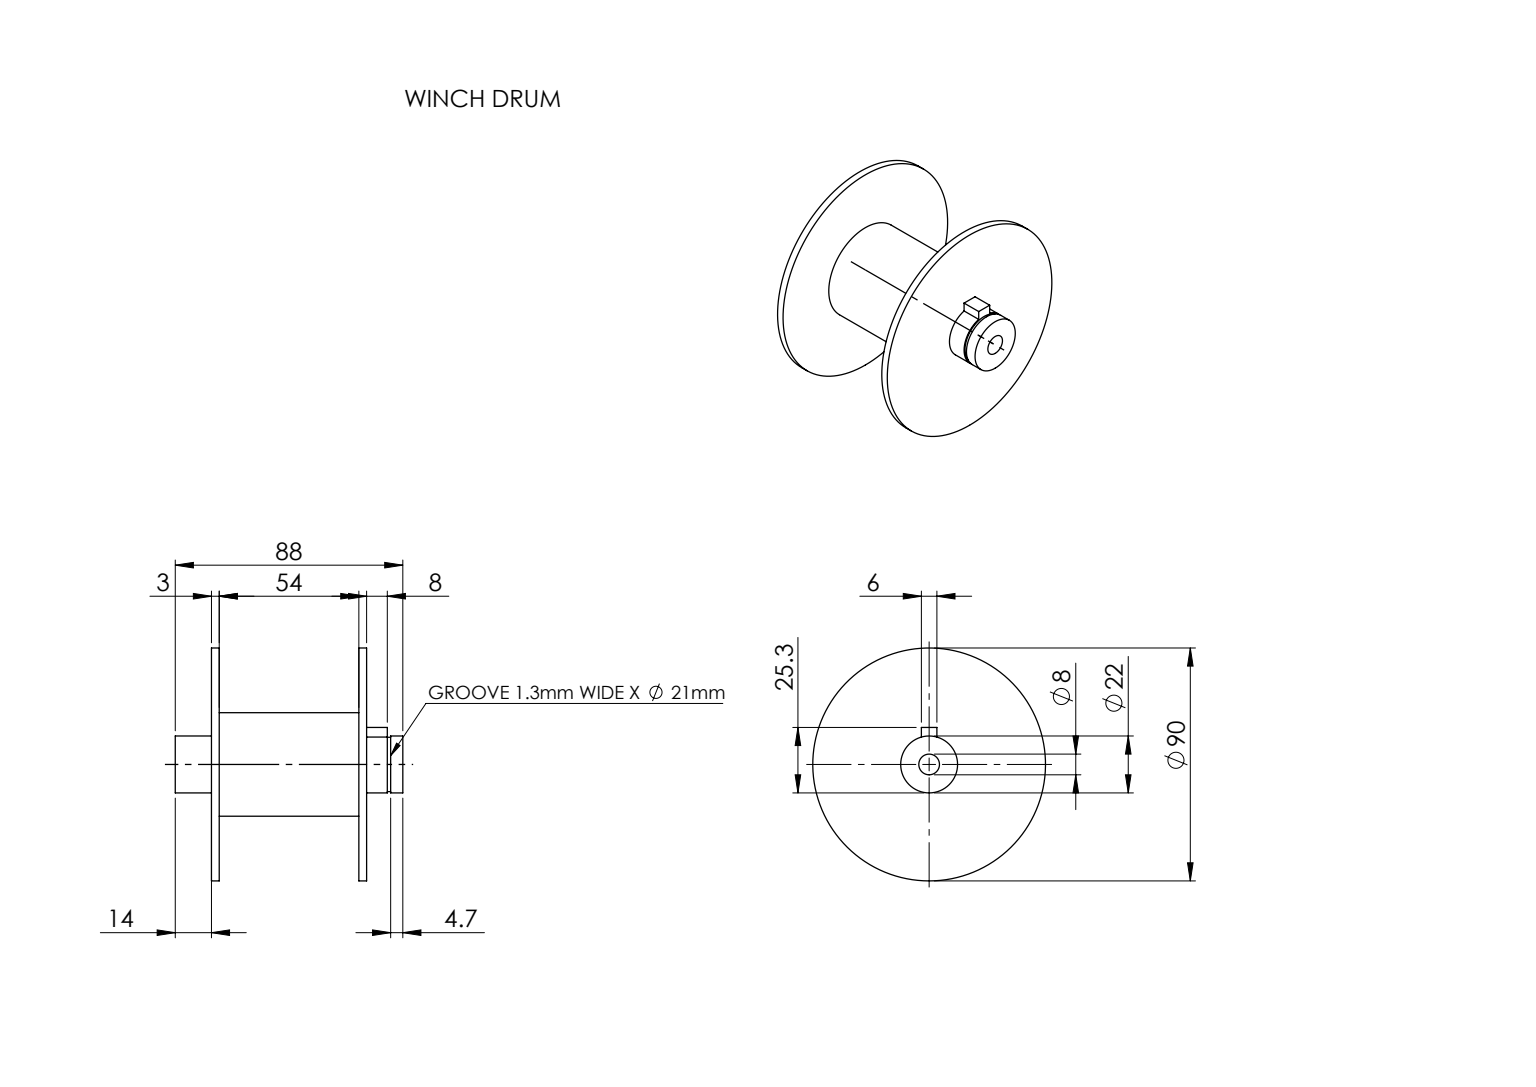
ISO-10303-21;
HEADER;
FILE_DESCRIPTION (('STEP AP214'),
    '1' );
FILE_NAME ('winch drum.step',
    '2026-09-28T15:49:00',
    ( '' ),
    ( '' ),
    'SwSTEP 2.0',
    'SolidWorks 2026',
    '' );
FILE_SCHEMA (( 'AUTOMOTIVE_DESIGN' ));
ENDSEC;

DATA;
#34=EDGE_CURVE ( 'NONE', #41, #24879, #23867, .T. ) ;
#41=VERTEX_POINT ( 'NONE', #30237 ) ;
#61=PRODUCT_DEFINITION_CONTEXT ( 'detailed design', #10343, 'design' ) ;
#131=DIRECTION ( 'NONE',  ( 3.154042683594195121E-16, -1.000000000000000000, 0.000000000000000000 ) ) ;
#150=CIRCLE ( 'NONE', #20253, 10.49999999999999645 ) ;
#165=EDGE_LOOP ( 'NONE', ( #34019, #14736, #9837, #7104, #34372 ) ) ;
#233=DIRECTION ( 'NONE',  ( 0.000000000000000000, 0.000000000000000000, -1.000000000000000000 ) ) ;
#284=CARTESIAN_POINT ( 'NONE',  ( 29.99999999999999289, 1.244980450007031636E-14, -3.000000000000002665 ) ) ;
#310=VECTOR ( 'NONE', #1724, 1000.000000000000000 ) ;
#429=DIRECTION ( 'NONE',  ( 0.000000000000000000, -1.000000000000000000, 0.000000000000000000 ) ) ;
#534=CYLINDRICAL_SURFACE ( 'NONE', #32662, 44.99999999999999289 ) ;
#567=ORIENTED_EDGE ( 'NONE', *, *, #16616, .F. ) ;
#653=CARTESIAN_POINT ( 'NONE',  ( 38.00000000000000000, -10.99999999999999112, 0.000000000000000000 ) ) ;
#680=DIRECTION ( 'NONE',  ( 1.000000000000000000, 1.836970198721029934E-16, 0.000000000000000000 ) ) ;
#700=DIRECTION ( 'NONE',  ( 1.541976423090495387E-16, -1.000000000000000000, 0.000000000000000000 ) ) ;
#729=ORIENTED_EDGE ( 'NONE', *, *, #32592, .F. ) ;
#737=CIRCLE ( 'NONE', #20844, 44.99999999999999289 ) ;
#790=DIRECTION ( 'NONE',  ( 1.734723475976807341E-16, -1.000000000000000000, 0.000000000000000000 ) ) ;
#808=DIRECTION ( 'NONE',  ( 1.000000000000000000, 1.836970198721029934E-16, 0.000000000000000000 ) ) ;
#834=DIRECTION ( 'NONE',  ( 1.734723475976807834E-16, -1.000000000000000000, 0.000000000000000000 ) ) ;
#871=ADVANCED_FACE ( 'NONE', ( #21988 ), #35173, .F. ) ;
#894=FACE_OUTER_BOUND ( 'NONE', #8453, .T. ) ;
#910=DIRECTION ( 'NONE',  ( -1.836970198721029934E-16, 1.000000000000000000, 0.000000000000000000 ) ) ;
#1012=CARTESIAN_POINT ( 'NONE',  ( -22.99999999999999645, 3.857637417314163478E-15, 0.000000000000000000 ) ) ;
#1033=AXIS2_PLACEMENT_3D ( 'NONE', #11770, #24941, #790 ) ;
#1034=CARTESIAN_POINT ( 'NONE',  ( 26.99999999999999645, 1.304248841091931221E-14, 0.000000000000000000 ) ) ;
#1094=CARTESIAN_POINT ( 'NONE',  ( 44.00000000000000000, 1.616533774874506480E-14, 0.000000000000000000 ) ) ;
#1149=DIRECTION ( 'NONE',  ( 1.836970198721029934E-16, -1.000000000000000000, 0.000000000000000000 ) ) ;
#1170=ADVANCED_FACE ( 'NONE', ( #1274 ), #14768, .T. ) ;
#1183=PRODUCT_DEFINITION_SHAPE ( 'NONE', 'NONE',  #8382 ) ;
#1274=FACE_OUTER_BOUND ( 'NONE', #3438, .T. ) ;
#1275=VERTEX_POINT ( 'NONE', #9555 ) ;
#1338=ORIENTED_EDGE ( 'NONE', *, *, #30581, .T. ) ;
#1358=( NAMED_UNIT ( * ) SI_UNIT ( $, .STERADIAN. ) SOLID_ANGLE_UNIT ( ) );
#1382=SURFACE_SIDE_STYLE ('',( #4458 ) ) ;
#1393=FACE_BOUND ( 'NONE', #12136, .T. ) ;
#1406=DIRECTION ( 'NONE',  ( -1.000000000000000000, -1.836970198721029934E-16, 0.000000000000000000 ) ) ;
#1491=EDGE_CURVE ( 'NONE', #24853, #25123, #7740, .T. ) ;
#1513=ORIENTED_EDGE ( 'NONE', *, *, #21110, .T. ) ;
#1516=AXIS2_PLACEMENT_3D ( 'NONE', #30895, #33779, #6052 ) ;
#1523=AXIS2_PLACEMENT_3D ( 'NONE', #1094, #7014, #25409 ) ;
#1528=LINE ( 'NONE', #4424, #20843 ) ;
#1550=DIRECTION ( 'NONE',  ( 0.000000000000000000, 1.000000000000000000, 0.000000000000000000 ) ) ;
#1553=VECTOR ( 'NONE', #30936, 1000.000000000000000 ) ;
#1561=AXIS2_PLACEMENT_3D ( 'NONE', #12165, #14670, #23140 ) ;
#1629=CARTESIAN_POINT ( 'NONE',  ( 39.30000000000000426, 7.219292880973646134E-15, 0.000000000000000000 ) ) ;
#1652=AXIS2_PLACEMENT_3D ( 'NONE', #17026, #25693, #30390 ) ;
#1669=ORIENTED_EDGE ( 'NONE', *, *, #12636, .T. ) ;
#1724=DIRECTION ( 'NONE',  ( -1.836970198721029934E-16, 1.000000000000000000, 0.000000000000000000 ) ) ;
#1739=( NAMED_UNIT ( * ) PLANE_ANGLE_UNIT ( ) SI_UNIT ( $, .RADIAN. ) );
#1752=PLANE ( 'NONE',  #4563 ) ;
#1779=VERTEX_POINT ( 'NONE', #25208 ) ;
#1781=PRODUCT ( 'winch drum', 'winch drum', '', ( #12191 ) ) ;
#1835=AXIS2_PLACEMENT_3D ( 'NONE', #34697, #7844, #15755 ) ;
#1882=VERTEX_POINT ( 'NONE', #12759 ) ;
#1918=LINE ( 'NONE', #4971, #30830 ) ;
#1947=DIRECTION ( 'NONE',  ( -1.000000000000000000, -1.836970198721029934E-16, -0.000000000000000000 ) ) ;
#2037=AXIS2_PLACEMENT_3D ( 'NONE', #13813, #8223, #5538 ) ;
#2085=DIRECTION ( 'NONE',  ( 0.000000000000000000, -1.000000000000000000, 0.000000000000000000 ) ) ;
#2092=AXIS2_PLACEMENT_3D ( 'NONE', #17775, #33632, #17418 ) ;
#2113=ORIENTED_EDGE ( 'NONE', *, *, #8351, .T. ) ;
#2141=AXIS2_PLACEMENT_3D ( 'NONE', #4828, #4661, #4297 ) ;
#2168=ORIENTED_EDGE ( 'NONE', *, *, #34254, .F. ) ;
#2203=CARTESIAN_POINT ( 'NONE',  ( -44.00000000000000000, 11.00000000000000000, 1.347111479062088405E-15 ) ) ;
#2246=ORIENTED_EDGE ( 'NONE', *, *, #21285, .T. ) ;
#2279=CIRCLE ( 'NONE', #10897, 10.49999999999999645 ) ;
#2280=DIRECTION ( 'NONE',  ( 3.154042683594195121E-16, -1.000000000000000000, 0.000000000000000000 ) ) ;
#2333=ORIENTED_EDGE ( 'NONE', *, *, #28174, .T. ) ;
#2369=ORIENTED_EDGE ( 'NONE', *, *, #34308, .T. ) ;
#2446=LINE ( 'NONE', #21493, #310 ) ;
#2540=ADVANCED_FACE ( 'NONE', ( #10376 ), #24072, .F. ) ;
#2629=DIRECTION ( 'NONE',  ( -1.000000000000000000, -1.836970198721029934E-16, -0.000000000000000000 ) ) ;
#2634=AXIS2_PLACEMENT_3D ( 'NONE', #1034, #14505, #834 ) ;
#2664=CYLINDRICAL_SURFACE ( 'NONE', #12460, 45.00000000000000000 ) ;
#2699=ORIENTED_EDGE ( 'NONE', *, *, #1491, .F. ) ;
#2713=SURFACE_STYLE_USAGE ( .BOTH. , #16349 ) ;
#2723=CARTESIAN_POINT ( 'NONE',  ( 38.00000000000000000, 14.30000000000001492, -3.000000000000002665 ) ) ;
#2724=VECTOR ( 'NONE', #29273, 1000.000000000000000 ) ;
#2736=EDGE_LOOP ( 'NONE', ( #16922, #13731, #9263, #6785 ) ) ;
#2765=DIRECTION ( 'NONE',  ( 0.000000000000000000, -1.000000000000000000, 0.000000000000000000 ) ) ;
#2786=DIRECTION ( 'NONE',  ( -1.000000000000000000, -1.836970198721029934E-16, -0.000000000000000000 ) ) ;
#2805=FACE_BOUND ( 'NONE', #34964, .T. ) ;
#2840=VECTOR ( 'NONE', #7984, 1000.000000000000000 ) ;
#2981=DIRECTION ( 'NONE',  ( 1.000000000000000000, 1.836970198721029934E-16, 0.000000000000000000 ) ) ;
#2988=CARTESIAN_POINT ( 'NONE',  ( -44.00199999999999534, 14.29999999999999893, 3.000000000000002665 ) ) ;
#2989=EDGE_LOOP ( 'NONE', ( #17604, #28300, #12736, #33040 ) ) ;
#2998=ORIENTED_EDGE ( 'NONE', *, *, #27190, .T. ) ;
#3023=FACE_OUTER_BOUND ( 'NONE', #30000, .T. ) ;
#3043=AXIS2_PLACEMENT_3D ( 'NONE', #26710, #10316, #29585 ) ;
#3045=VECTOR ( 'NONE', #27840, 1000.000000000000000 ) ;
#3108=EDGE_LOOP ( 'NONE', ( #13392, #17439, #19443, #29588 ) ) ;
#3152=DIRECTION ( 'NONE',  ( 1.541976423090495140E-16, -1.000000000000000000, 0.000000000000000000 ) ) ;
#3154=CARTESIAN_POINT ( 'NONE',  ( 26.99999999999999289, 20.00000000000000711, 2.449293598294706513E-15 ) ) ;
#3188=CARTESIAN_POINT ( 'NONE',  ( -44.00000000000000000, 3.999999999999998224, 4.898587196589410857E-16 ) ) ;
#3250=FACE_OUTER_BOUND ( 'NONE', #5593, .T. ) ;
#3291=ORIENTED_EDGE ( 'NONE', *, *, #27599, .F. ) ;
#3297=ORIENTED_EDGE ( 'NONE', *, *, #17207, .T. ) ;
#3351=ORIENTED_EDGE ( 'NONE', *, *, #23483, .T. ) ;
#3383=DIRECTION ( 'NONE',  ( -1.000000000000000000, -1.836970198721029934E-16, -0.000000000000000000 ) ) ;
#3438=EDGE_LOOP ( 'NONE', ( #15500, #5981, #28662, #25374 ) ) ;
#3454=CYLINDRICAL_SURFACE ( 'NONE', #10008, 10.49999999999999645 ) ;
#3478=CARTESIAN_POINT ( 'NONE',  ( 38.00000000000000000, 14.30000000000001492, 3.000000000000002665 ) ) ;
#3508=FACE_OUTER_BOUND ( 'NONE', #17433, .T. ) ;
#3627=ORIENTED_EDGE ( 'NONE', *, *, #21126, .T. ) ;
#3654=FACE_OUTER_BOUND ( 'NONE', #2736, .T. ) ;
#3662=CARTESIAN_POINT ( 'NONE',  ( 38.00000000000000000, 6.980486755139912911E-15, 0.000000000000000000 ) ) ;
#3675=DIRECTION ( 'NONE',  ( -1.000000000000000000, -1.836970198721029934E-16, -0.000000000000000000 ) ) ;
#3697=EDGE_CURVE ( 'NONE', #4637, #10821, #30092, .T. ) ;
#3761=DIRECTION ( 'NONE',  ( -1.000000000000000000, -1.836970198721029934E-16, -0.000000000000000000 ) ) ;
#3841=DIRECTION ( 'NONE',  ( 0.000000000000000000, -1.000000000000000000, 0.000000000000000000 ) ) ;
#3861=DIRECTION ( 'NONE',  ( -1.000000000000000000, -1.836970198721029934E-16, 0.000000000000000000 ) ) ;
#3897=FILL_AREA_STYLE ('',( #28549 ) ) ;
#3991=CARTESIAN_POINT ( 'NONE',  ( -22.99999999999999289, -12.99999999999999645, 0.000000000000000000 ) ) ;
#4015=VECTOR ( 'NONE', #13104, 1000.000000000000000 ) ;
#4034=DIRECTION ( 'NONE',  ( 0.000000000000000000, 1.000000000000000000, 0.000000000000000000 ) ) ;
#4126=LINE ( 'NONE', #34003, #8071 ) ;
#4174=ORIENTED_EDGE ( 'NONE', *, *, #21174, .F. ) ;
#4193=VERTEX_POINT ( 'NONE', #6439 ) ;
#4203=CARTESIAN_POINT ( 'NONE',  ( -23.00000000000000355, 3.857637417314161900E-15, 0.000000000000000000 ) ) ;
#4275=ORIENTED_EDGE ( 'NONE', *, *, #12327, .F. ) ;
#4293=AXIS2_PLACEMENT_3D ( 'NONE', #21671, #10888, #910 ) ;
#4297=DIRECTION ( 'NONE',  ( 0.000000000000000000, 1.000000000000000000, 0.000000000000000000 ) ) ;
#4344=EDGE_LOOP ( 'NONE', ( #19756, #2369 ) ) ;
#4424=CARTESIAN_POINT ( 'NONE',  ( -43.99999999999999289, -19.99999999999999645, 0.000000000000000000 ) ) ;
#4458=SURFACE_STYLE_FILL_AREA ( #34511 ) ;
#4460=VECTOR ( 'NONE', #33523, 1000.000000000000000 ) ;
#4471=CYLINDRICAL_SURFACE ( 'NONE', #34358, 19.99999999999999645 ) ;
#4559=FACE_OUTER_BOUND ( 'NONE', #9559, .T. ) ;
#4563=AXIS2_PLACEMENT_3D ( 'NONE', #17575, #15052, #6787 ) ;
#4584=LINE ( 'NONE', #9783, #27949 ) ;
#4587=CIRCLE ( 'NONE', #24693, 3.999999999999996447 ) ;
#4588=DIRECTION ( 'NONE',  ( 1.836970198721029934E-16, -1.000000000000000000, 0.000000000000000000 ) ) ;
#4621=CARTESIAN_POINT ( 'NONE',  ( 38.00000000000000000, 10.58300524425836642, 3.000000000000002665 ) ) ;
#4634=EDGE_LOOP ( 'NONE', ( #29738, #4894, #23434, #33229 ) ) ;
#4637=VERTEX_POINT ( 'NONE', #29264 ) ;
#4650=ADVANCED_FACE ( 'NONE', ( #9987 ), #26929, .T. ) ;
#4661=DIRECTION ( 'NONE',  ( 1.000000000000000000, 1.836970198721029934E-16, 0.000000000000000000 ) ) ;
#4669=MECHANICAL_DESIGN_GEOMETRIC_PRESENTATION_REPRESENTATION('',(#24779),#25931);
#4740=ADVANCED_FACE ( 'NONE', ( #22679 ), #3454, .T. ) ;
#4771=VERTEX_POINT ( 'NONE', #30980 ) ;
#4806=VERTEX_POINT ( 'NONE', #14578 ) ;
#4814=ADVANCED_FACE ( 'NONE', ( #2805, #25590 ), #16254, .F. ) ;
#4828=CARTESIAN_POINT ( 'NONE',  ( 38.00000000000000000, 6.980486755139912911E-15, 0.000000000000000000 ) ) ;
#4894=ORIENTED_EDGE ( 'NONE', *, *, #17863, .T. ) ;
#4911=CYLINDRICAL_SURFACE ( 'NONE', #19404, 10.99999999999999289 ) ;
#4971=CARTESIAN_POINT ( 'NONE',  ( -44.00000000000000000, -3.999999999999993339, 0.000000000000000000 ) ) ;
#4993=AXIS2_PLACEMENT_3D ( 'NONE', #10499, #34818, #15704 ) ;
#4994=VECTOR ( 'NONE', #20065, 1000.000000000000000 ) ;
#5001=DIRECTION ( 'NONE',  ( 1.734723475976807341E-16, -1.000000000000000000, 0.000000000000000000 ) ) ;
#5047=CIRCLE ( 'NONE', #25165, 10.49999999999999645 ) ;
#5085=DIRECTION ( 'NONE',  ( -1.000000000000000000, -1.836970198721029934E-16, -0.000000000000000000 ) ) ;
#5105=CARTESIAN_POINT ( 'NONE',  ( 44.00000000000000000, 11.00000000000001066, 0.000000000000000000 ) ) ;
#5217=VERTEX_POINT ( 'NONE', #33628 ) ;
#5273=ORIENTED_EDGE ( 'NONE', *, *, #22487, .F. ) ;
#5275=DIRECTION ( 'NONE',  ( -1.000000000000000000, -1.836970198721029934E-16, -0.000000000000000000 ) ) ;
#5363=EDGE_CURVE ( 'NONE', #34165, #17302, #12212, .T. ) ;
#5372=ORIENTED_EDGE ( 'NONE', *, *, #16356, .T. ) ;
#5432=VERTEX_POINT ( 'NONE', #28775 ) ;
#5465=VERTEX_POINT ( 'NONE', #6445 ) ;
#5487=PLANE ( 'NONE',  #26590 ) ;
#5500=PLANE ( 'NONE',  #15316 ) ;
#5538=DIRECTION ( 'NONE',  ( 2.668805347656627171E-16, -1.000000000000000000, 0.000000000000000000 ) ) ;
#5565=CIRCLE ( 'NONE', #1523, 10.99999999999999467 ) ;
#5593=EDGE_LOOP ( 'NONE', ( #31361, #24336, #6274, #32233 ) ) ;
#5647=LINE ( 'NONE', #3478, #11531 ) ;
#5654=LINE ( 'NONE', #21657, #2840 ) ;
#5685=EDGE_LOOP ( 'NONE', ( #32579, #12274 ) ) ;
#5699=AXIS2_PLACEMENT_3D ( 'NONE', #26558, #26733, #26016 ) ;
#5702=DIRECTION ( 'NONE',  ( 0.000000000000000000, -1.000000000000000000, 0.000000000000000000 ) ) ;
#5768=ADVANCED_FACE ( 'NONE', ( #14318, #33413 ), #19884, .F. ) ;
#5896=VECTOR ( 'NONE', #12868, 1000.000000000000000 ) ;
#5905=AXIS2_PLACEMENT_3D ( 'NONE', #5105, #10852, #16398 ) ;
#5924=ORIENTED_EDGE ( 'NONE', *, *, #14525, .T. ) ;
#5928=ORIENTED_EDGE ( 'NONE', *, *, #8757, .T. ) ;
#5979=LINE ( 'NONE', #30476, #18798 ) ;
#5981=ORIENTED_EDGE ( 'NONE', *, *, #15173, .T. ) ;
#5987=CARTESIAN_POINT ( 'NONE',  ( 39.30000000000000426, 7.219292880973646134E-15, 0.000000000000000000 ) ) ;
#6020=LINE ( 'NONE', #33382, #33730 ) ;
#6052=DIRECTION ( 'NONE',  ( 1.541976423090495387E-16, -1.000000000000000000, 0.000000000000000000 ) ) ;
#6113=VERTEX_POINT ( 'NONE', #4621 ) ;
#6114=CARTESIAN_POINT ( 'NONE',  ( 27.00000000000000355, 45.00000000000000711, 5.510910596163087978E-15 ) ) ;
#6123=EDGE_CURVE ( 'NONE', #29440, #10721, #2446, .T. ) ;
#6165=EDGE_LOOP ( 'NONE', ( #3297, #7262 ) ) ;
#6193=FACE_OUTER_BOUND ( 'NONE', #7487, .T. ) ;
#6223=DIRECTION ( 'NONE',  ( 0.000000000000000000, 0.000000000000000000, -1.000000000000000000 ) ) ;
#6274=ORIENTED_EDGE ( 'NONE', *, *, #15016, .T. ) ;
#6282=EDGE_LOOP ( 'NONE', ( #15476, #24782 ) ) ;
#6294=CARTESIAN_POINT ( 'NONE',  ( 38.00000000000000000, 10.50000000000000355, 1.285879139104720436E-15 ) ) ;
#6357=CARTESIAN_POINT ( 'NONE',  ( -44.00000000000000000, 0.000000000000000000, 0.000000000000000000 ) ) ;
#6437=ADVANCED_FACE ( 'NONE', ( #6193, #34268 ), #25825, .T. ) ;
#6439=CARTESIAN_POINT ( 'NONE',  ( -44.00000000000000000, 4.000000000000000000, 4.898587196589411843E-16 ) ) ;
#6445=CARTESIAN_POINT ( 'NONE',  ( 23.00000000000000711, -3.999999999999980904, 0.000000000000000000 ) ) ;
#6486=CARTESIAN_POINT ( 'NONE',  ( -23.00000000000000355, -3.999999999999993339, 0.000000000000000000 ) ) ;
#6490=EDGE_LOOP ( 'NONE', ( #23871, #9576 ) ) ;
#6714=ORIENTED_EDGE ( 'NONE', *, *, #22194, .T. ) ;
#6734=AXIS2_PLACEMENT_3D ( 'NONE', #8385, #19368, #5702 ) ;
#6736=ORIENTED_EDGE ( 'NONE', *, *, #26085, .T. ) ;
#6760=DIRECTION ( 'NONE',  ( 0.000000000000000000, -1.000000000000000000, 0.000000000000000000 ) ) ;
#6785=ORIENTED_EDGE ( 'NONE', *, *, #32376, .F. ) ;
#6787=DIRECTION ( 'NONE',  ( -1.000000000000000000, 0.000000000000000000, -0.000000000000000000 ) ) ;
#6862=APPLICATION_CONTEXT ( 'automotive_design' ) ;
#6906=ORIENTED_EDGE ( 'NONE', *, *, #28725, .F. ) ;
#6913=ORIENTED_EDGE ( 'NONE', *, *, #19760, .F. ) ;
#6955=( NAMED_UNIT ( * ) SI_UNIT ( $, .STERADIAN. ) SOLID_ANGLE_UNIT ( ) );
#7014=DIRECTION ( 'NONE',  ( -1.000000000000000000, -1.836970198721029934E-16, -0.000000000000000000 ) ) ;
#7104=ORIENTED_EDGE ( 'NONE', *, *, #33042, .T. ) ;
#7121=ORIENTED_EDGE ( 'NONE', *, *, #32873, .T. ) ;
#7144=CARTESIAN_POINT ( 'NONE',  ( 38.00000000000000000, 6.980486755139912911E-15, 0.000000000000000000 ) ) ;
#7206=CIRCLE ( 'NONE', #2634, 19.99999999999999289 ) ;
#7229=ORIENTED_EDGE ( 'NONE', *, *, #15016, .F. ) ;
#7262=ORIENTED_EDGE ( 'NONE', *, *, #34832, .T. ) ;
#7467=VECTOR ( 'NONE', #13834, 1000.000000000000000 ) ;
#7487=EDGE_LOOP ( 'NONE', ( #2998, #1669 ) ) ;
#7497=LINE ( 'NONE', #10562, #4015 ) ;
#7612=AXIS2_PLACEMENT_3D ( 'NONE', #25114, #30168, #19854 ) ;
#7675=CARTESIAN_POINT ( 'NONE',  ( 38.00000000000000000, 6.980486755139912911E-15, 0.000000000000000000 ) ) ;
#7696=CIRCLE ( 'NONE', #27279, 10.99999999999999822 ) ;
#7722=CARTESIAN_POINT ( 'NONE',  ( 22.99999999999999289, 1.230770033143089817E-14, 0.000000000000000000 ) ) ;
#7740=LINE ( 'NONE', #2203, #23211 ) ;
#7820=CIRCLE ( 'NONE', #34365, 45.00000000000000000 ) ;
#7830=CIRCLE ( 'NONE', #1516, 44.99999999999999289 ) ;
#7831=ORIENTED_EDGE ( 'NONE', *, *, #9791, .T. ) ;
#7843=CIRCLE ( 'NONE', #8993, 45.00000000000000000 ) ;
#7844=DIRECTION ( 'NONE',  ( -1.000000000000000000, -1.836970198721029934E-16, -0.000000000000000000 ) ) ;
#7850=CARTESIAN_POINT ( 'NONE',  ( 44.00000000000000000, 4.000000000000010658, 4.898587196589409870E-16 ) ) ;
#7885=LINE ( 'NONE', #16153, #28240 ) ;
#7920=EDGE_LOOP ( 'NONE', ( #20972, #2333 ) ) ;
#7984=DIRECTION ( 'NONE',  ( -1.000000000000000000, -1.836970198721029934E-16, -0.000000000000000000 ) ) ;
#7986=CARTESIAN_POINT ( 'NONE',  ( -44.00000000000000000, 0.000000000000000000, 0.000000000000000000 ) ) ;
#8004=PLANE ( 'NONE',  #29158 ) ;
#8063=CYLINDRICAL_SURFACE ( 'NONE', #27127, 10.99999999999999289 ) ;
#8064=ORIENTED_EDGE ( 'NONE', *, *, #32592, .T. ) ;
#8071=VECTOR ( 'NONE', #17588, 1000.000000000000000 ) ;
#8223=DIRECTION ( 'NONE',  ( -1.000000000000000000, -1.836970198721029934E-16, -0.000000000000000000 ) ) ;
#8229=EDGE_CURVE ( 'NONE', #4771, #35305, #5565, .T. ) ;
#8351=EDGE_CURVE ( 'NONE', #5217, #15608, #9723, .T. ) ;
#8382=PRODUCT_DEFINITION ( 'UNKNOWN', '', #32202, #61 ) ;
#8385=CARTESIAN_POINT ( 'NONE',  ( -44.00000000000000000, 0.000000000000000000, 0.000000000000000000 ) ) ;
#8425=AXIS2_PLACEMENT_3D ( 'NONE', #15592, #1947, #5001 ) ;
#8453=EDGE_LOOP ( 'NONE', ( #17555, #18112, #6736, #22714 ) ) ;
#8539=DIRECTION ( 'NONE',  ( 1.836970198721029934E-16, -1.000000000000000000, 0.000000000000000000 ) ) ;
#8569=CARTESIAN_POINT ( 'NONE',  ( -27.00000000000000000, 45.00000000000000000, 0.000000000000000000 ) ) ;
#8574=CYLINDRICAL_SURFACE ( 'NONE', #18688, 11.00000000000000000 ) ;
#8624=ORIENTED_EDGE ( 'NONE', *, *, #35054, .T. ) ;
#8678=CARTESIAN_POINT ( 'NONE',  ( 44.00000000000000000, -3.999999999999977351, 0.000000000000000000 ) ) ;
#8702=DIRECTION ( 'NONE',  ( -1.000000000000000000, -1.836970198721029934E-16, -0.000000000000000000 ) ) ;
#8747=ADVANCED_FACE ( 'NONE', ( #14710, #19922 ), #28771, .F. ) ;
#8757=EDGE_CURVE ( 'NONE', #10721, #15971, #20106, .T. ) ;
#8873=EDGE_CURVE ( 'NONE', #6113, #34165, #28563, .T. ) ;
#8923=VERTEX_POINT ( 'NONE', #32182 ) ;
#8963=CARTESIAN_POINT ( 'NONE',  ( -26.99999999999999289, 3.122849337825751800E-15, 0.000000000000000000 ) ) ;
#8993=AXIS2_PLACEMENT_3D ( 'NONE', #8963, #3761, #20466 ) ;
#9003=CIRCLE ( 'NONE', #4993, 3.999999999999996447 ) ;
#9005=CIRCLE ( 'NONE', #32585, 10.99999999999999822 ) ;
#9012=EDGE_CURVE ( 'NONE', #31306, #31368, #16489, .T. ) ;
#9062=CYLINDRICAL_SURFACE ( 'NONE', #15065, 44.99999999999999289 ) ;
#9073=ORIENTED_EDGE ( 'NONE', *, *, #28700, .F. ) ;
#9091=ADVANCED_BREP_SHAPE_REPRESENTATION ( '', ( #22543, #21307 ), #35148 ) ;
#9144=CARTESIAN_POINT ( 'NONE',  ( 39.30000000000000426, 7.219292880973646134E-15, 0.000000000000000000 ) ) ;
#9174=DIRECTION ( 'NONE',  ( 0.000000000000000000, -1.000000000000000000, 0.000000000000000000 ) ) ;
#9222=ADVANCED_FACE ( 'NONE', ( #33068 ), #33245, .T. ) ;
#9263=ORIENTED_EDGE ( 'NONE', *, *, #16971, .T. ) ;
#9280=CARTESIAN_POINT ( 'NONE',  ( -44.00000000000000711, 45.00000000000000000, 5.510910596163089556E-15 ) ) ;
#9295=DIRECTION ( 'NONE',  ( 1.541976423090495140E-16, -1.000000000000000000, 0.000000000000000000 ) ) ;
#9327=FACE_OUTER_BOUND ( 'NONE', #15946, .T. ) ;
#9351=ORIENTED_EDGE ( 'NONE', *, *, #21110, .F. ) ;
#9377=VERTEX_POINT ( 'NONE', #27276 ) ;
#9470=LINE ( 'NONE', #34147, #30884 ) ;
#9555=CARTESIAN_POINT ( 'NONE',  ( 22.99999999999999645, -12.99999999999998224, 0.000000000000000000 ) ) ;
#9559=EDGE_LOOP ( 'NONE', ( #24810, #20692, #25514, #4275 ) ) ;
#9572=CIRCLE ( 'NONE', #13585, 45.00000000000000000 ) ;
#9576=ORIENTED_EDGE ( 'NONE', *, *, #33921, .F. ) ;
#9599=CIRCLE ( 'NONE', #1561, 3.999999999999994227 ) ;
#9642=AXIS2_PLACEMENT_3D ( 'NONE', #13544, #5275, #15868 ) ;
#9653=DIRECTION ( 'NONE',  ( -1.000000000000000000, -1.836970198721029934E-16, -0.000000000000000000 ) ) ;
#9709=EDGE_LOOP ( 'NONE', ( #5273, #6714, #20331, #18873 ) ) ;
#9723=LINE ( 'NONE', #33665, #19972 ) ;
#9783=CARTESIAN_POINT ( 'NONE',  ( 39.30000000000000426, 10.50000000000000355, 1.285879139104720436E-15 ) ) ;
#9791=EDGE_CURVE ( 'NONE', #4806, #5465, #13688, .T. ) ;
#9805=DIRECTION ( 'NONE',  ( -1.000000000000000000, -1.836970198721029934E-16, -0.000000000000000000 ) ) ;
#9837=ORIENTED_EDGE ( 'NONE', *, *, #24243, .T. ) ;
#9878=EDGE_LOOP ( 'NONE', ( #35020, #27480 ) ) ;
#9920=CARTESIAN_POINT ( 'NONE',  ( 38.00000000000000000, 14.30000000000001492, 3.000000000000002665 ) ) ;
#9987=FACE_OUTER_BOUND ( 'NONE', #28604, .T. ) ;
#10008=AXIS2_PLACEMENT_3D ( 'NONE', #28285, #24389, #19319 ) ;
#10013=FILL_AREA_STYLE_COLOUR ( '', #32253 ) ;
#10102=DIRECTION ( 'NONE',  ( 0.000000000000000000, -1.000000000000000000, 0.000000000000000000 ) ) ;
#10144=VERTEX_POINT ( 'NONE', #25238 ) ;
#10200=( LENGTH_UNIT ( ) NAMED_UNIT ( * ) SI_UNIT ( .MILLI., .METRE. ) );
#10215=FACE_OUTER_BOUND ( 'NONE', #2989, .T. ) ;
#10234=CIRCLE ( 'NONE', #1033, 19.99999999999999645 ) ;
#10259=LINE ( 'NONE', #19050, #20090 ) ;
#10316=DIRECTION ( 'NONE',  ( -1.000000000000000000, -1.836970198721029934E-16, -0.000000000000000000 ) ) ;
#10343=APPLICATION_CONTEXT ( 'automotive_design' ) ;
#10376=FACE_OUTER_BOUND ( 'NONE', #12226, .T. ) ;
#10421=CARTESIAN_POINT ( 'NONE',  ( -30.00000000000000000, 2.571758278209441661E-15, 0.000000000000000000 ) ) ;
#10429=CARTESIAN_POINT ( 'NONE',  ( -26.99999999999999645, 20.00000000000000000, 2.449293598294706119E-15 ) ) ;
#10499=CARTESIAN_POINT ( 'NONE',  ( -23.00000000000000355, 3.857637417314161900E-15, 0.000000000000000000 ) ) ;
#10562=CARTESIAN_POINT ( 'NONE',  ( -44.00000000000000000, -3.999999999999998224, 0.000000000000000000 ) ) ;
#10598=CARTESIAN_POINT ( 'NONE',  ( -44.00000000000000000, 0.000000000000000000, 0.000000000000000000 ) ) ;
#10712=CIRCLE ( 'NONE', #24520, 44.99999999999999289 ) ;
#10721=VERTEX_POINT ( 'NONE', #24402 ) ;
#10744=CARTESIAN_POINT ( 'NONE',  ( 38.00000000000000000, 1.391938065904714129E-14, 3.000000000000002665 ) ) ;
#10752=FACE_OUTER_BOUND ( 'NONE', #9709, .T. ) ;
#10784=ADVANCED_FACE ( 'NONE', ( #22043 ), #35389, .T. ) ;
#10821=VERTEX_POINT ( 'NONE', #27284 ) ;
#10852=DIRECTION ( 'NONE',  ( 1.000000000000000000, 1.836970198721029934E-16, 0.000000000000000000 ) ) ;
#10888=DIRECTION ( 'NONE',  ( 1.000000000000000000, 1.836970198721029934E-16, 0.000000000000000000 ) ) ;
#10897=AXIS2_PLACEMENT_3D ( 'NONE', #3662, #27793, #233 ) ;
#10904=CARTESIAN_POINT ( 'NONE',  ( -44.00000000000000711, 19.99999999999999645, 2.449293598294706119E-15 ) ) ;
#10914=( NAMED_UNIT ( * ) SI_UNIT ( $, .STERADIAN. ) SOLID_ANGLE_UNIT ( ) );
#11117=DIRECTION ( 'NONE',  ( 1.541976423090495387E-16, -1.000000000000000000, 0.000000000000000000 ) ) ;
#11180=DIRECTION ( 'NONE',  ( -1.000000000000000000, -1.836970198721029934E-16, -0.000000000000000000 ) ) ;
#11287=DIRECTION ( 'NONE',  ( -1.000000000000000000, -1.836970198721029934E-16, -0.000000000000000000 ) ) ;
#11383=ORIENTED_EDGE ( 'NONE', *, *, #31451, .F. ) ;
#11396=DIRECTION ( 'NONE',  ( 0.000000000000000000, 0.000000000000000000, -1.000000000000000000 ) ) ;
#11425=DIRECTION ( 'NONE',  ( 1.000000000000000000, 1.836970198721029934E-16, 0.000000000000000000 ) ) ;
#11445=DIRECTION ( 'NONE',  ( 0.000000000000000000, -1.000000000000000000, 0.000000000000000000 ) ) ;
#11455=DIRECTION ( 'NONE',  ( 1.836970198721029934E-16, -1.000000000000000000, 0.000000000000000000 ) ) ;
#11473=CARTESIAN_POINT ( 'NONE',  ( 30.00000000000000000, 14.30000000000001315, -3.000000000000002665 ) ) ;
#11531=VECTOR ( 'NONE', #11396, 1000.000000000000000 ) ;
#11563=LINE ( 'NONE', #22532, #4460 ) ;
#11566=ORIENTED_EDGE ( 'NONE', *, *, #27965, .F. ) ;
#11648=LINE ( 'NONE', #25354, #7467 ) ;
#11770=CARTESIAN_POINT ( 'NONE',  ( -26.99999999999999289, 3.122849337825751800E-15, 0.000000000000000000 ) ) ;
#11781=CYLINDRICAL_SURFACE ( 'NONE', #12798, 19.99999999999999645 ) ;
#11874=CYLINDRICAL_SURFACE ( 'NONE', #32735, 10.99999999999999289 ) ;
#11929=EDGE_CURVE ( 'NONE', #30594, #18020, #18488, .T. ) ;
#12013=EDGE_LOOP ( 'NONE', ( #2699, #16695, #7121, #20258 ) ) ;
#12016=CARTESIAN_POINT ( 'NONE',  ( -44.00000000000000000, -12.99999999999999822, 0.000000000000000000 ) ) ;
#12111=ADVANCED_FACE ( 'NONE', ( #21970 ), #29743, .F. ) ;
#12136=EDGE_LOOP ( 'NONE', ( #30615, #21113 ) ) ;
#12141=VERTEX_POINT ( 'NONE', #22805 ) ;
#12149=FACE_OUTER_BOUND ( 'NONE', #16778, .T. ) ;
#12165=CARTESIAN_POINT ( 'NONE',  ( 44.00000000000000000, 1.616533774874506480E-14, 0.000000000000000000 ) ) ;
#12171=CIRCLE ( 'NONE', #1835, 19.99999999999999289 ) ;
#12173=CARTESIAN_POINT ( 'NONE',  ( 39.30000000000000426, 7.219292880973646134E-15, 0.000000000000000000 ) ) ;
#12184=SURFACE_STYLE_USAGE ( .BOTH. , #1382 ) ;
#12185=COLOUR_RGB ( '', 0.66274510, 0.83137255, 0.94901961) ;
#12191=PRODUCT_CONTEXT ( 'NONE', #6862, 'mechanical' ) ;
#12193=VERTEX_POINT ( 'NONE', #26061 ) ;
#12200=PLANE ( 'NONE',  #29172 ) ;
#12212=LINE ( 'NONE', #34181, #13514 ) ;
#12226=EDGE_LOOP ( 'NONE', ( #9073, #28655, #7831, #30469 ) ) ;
#12255=ORIENTED_EDGE ( 'NONE', *, *, #12327, .T. ) ;
#12274=ORIENTED_EDGE ( 'NONE', *, *, #23106, .T. ) ;
#12327=EDGE_CURVE ( 'NONE', #1275, #24879, #12734, .T. ) ;
#12402=VECTOR ( 'NONE', #2629, 1000.000000000000000 ) ;
#12460=AXIS2_PLACEMENT_3D ( 'NONE', #13626, #24618, #17013 ) ;
#12636=EDGE_CURVE ( 'NONE', #1779, #1275, #15515, .T. ) ;
#12689=CARTESIAN_POINT ( 'NONE',  ( 39.30000000000000426, -10.49999999999999112, 0.000000000000000000 ) ) ;
#12702=( NAMED_UNIT ( * ) PLANE_ANGLE_UNIT ( ) SI_UNIT ( $, .RADIAN. ) );
#12706=CARTESIAN_POINT ( 'NONE',  ( -44.00000000000000000, 10.58300524425835398, 3.000000000000002665 ) ) ;
#12725=DIRECTION ( 'NONE',  ( 0.000000000000000000, 0.000000000000000000, 1.000000000000000000 ) ) ;
#12734=LINE ( 'NONE', #12016, #19100 ) ;
#12736=ORIENTED_EDGE ( 'NONE', *, *, #9012, .F. ) ;
#12759=CARTESIAN_POINT ( 'NONE',  ( 29.99999999999999645, 10.58300524425836819, -3.000000000000002665 ) ) ;
#12798=AXIS2_PLACEMENT_3D ( 'NONE', #17893, #33759, #14650 ) ;
#12868=DIRECTION ( 'NONE',  ( -1.000000000000000000, -1.836970198721030181E-16, 0.000000000000000000 ) ) ;
#13008=EDGE_CURVE ( 'NONE', #15971, #26642, #4126, .T. ) ;
#13018=ADVANCED_FACE ( 'NONE', ( #9327, #28598 ), #31475, .F. ) ;
#13093=ORIENTED_EDGE ( 'NONE', *, *, #31775, .F. ) ;
#13104=DIRECTION ( 'NONE',  ( -1.000000000000000000, -1.836970198721029934E-16, -0.000000000000000000 ) ) ;
#13106=CARTESIAN_POINT ( 'NONE',  ( -44.00000000000000000, 10.99999999999999289, 1.347111479062087616E-15 ) ) ;
#13139=DIRECTION ( 'NONE',  ( 0.000000000000000000, -1.000000000000000000, 0.000000000000000000 ) ) ;
#13291=CARTESIAN_POINT ( 'NONE',  ( 38.00000000000000000, -10.49999999999999112, 0.000000000000000000 ) ) ;
#13333=ADVANCED_FACE ( 'NONE', ( #10752 ), #2664, .T. ) ;
#13347=CARTESIAN_POINT ( 'NONE',  ( -26.99999999999998579, -45.00000000000000000, 0.000000000000000000 ) ) ;
#13392=ORIENTED_EDGE ( 'NONE', *, *, #34832, .F. ) ;
#13406=AXIS2_PLACEMENT_3D ( 'NONE', #1629, #22859, #20856 ) ;
#13412=CARTESIAN_POINT ( 'NONE',  ( -29.99999999999999645, 11.00000000000000000, 0.000000000000000000 ) ) ;
#13431=ORIENTED_EDGE ( 'NONE', *, *, #23483, .F. ) ;
#13514=VECTOR ( 'NONE', #31641, 1000.000000000000000 ) ;
#13515=DIRECTION ( 'NONE',  ( -1.000000000000000000, -1.836970198721029934E-16, -0.000000000000000000 ) ) ;
#13544=CARTESIAN_POINT ( 'NONE',  ( 23.00000000000000711, 1.230770033143090132E-14, 0.000000000000000000 ) ) ;
#13554=ORIENTED_EDGE ( 'NONE', *, *, #26376, .T. ) ;
#13555=DIRECTION ( 'NONE',  ( -1.000000000000000000, -1.836970198721029934E-16, 0.000000000000000000 ) ) ;
#13585=AXIS2_PLACEMENT_3D ( 'NONE', #16583, #27593, #24876 ) ;
#13626=CARTESIAN_POINT ( 'NONE',  ( -44.00000000000000000, 0.000000000000000000, 0.000000000000000000 ) ) ;
#13678=PRESENTATION_STYLE_ASSIGNMENT (( #2713 ) ) ;
#13688=CIRCLE ( 'NONE', #9642, 3.999999999999993339 ) ;
#13731=ORIENTED_EDGE ( 'NONE', *, *, #27965, .T. ) ;
#13773=CARTESIAN_POINT ( 'NONE',  ( -23.00000000000000000, 11.00000000000000000, 0.000000000000000000 ) ) ;
#13813=CARTESIAN_POINT ( 'NONE',  ( 22.99999999999999289, 1.230770033143089817E-14, 0.000000000000000000 ) ) ;
#13834=DIRECTION ( 'NONE',  ( -1.836970198721029934E-16, 1.000000000000000000, 0.000000000000000000 ) ) ;
#13889=EDGE_LOOP ( 'NONE', ( #35272, #2113, #27929, #7229 ) ) ;
#14080=DIRECTION ( 'NONE',  ( 1.000000000000000000, 1.836970198721029934E-16, 0.000000000000000000 ) ) ;
#14081=EDGE_CURVE ( 'NONE', #27829, #5217, #10712, .T. ) ;
#14138=CARTESIAN_POINT ( 'NONE',  ( 38.00000000000000000, 6.980486755139912911E-15, 0.000000000000000000 ) ) ;
#14208=ORIENTED_EDGE ( 'NONE', *, *, #17207, .F. ) ;
#14251=DIRECTION ( 'NONE',  ( 3.154042683594196600E-16, -1.000000000000000000, 0.000000000000000000 ) ) ;
#14271=EDGE_CURVE ( 'NONE', #8923, #32022, #7820, .T. ) ;
#14297=ORIENTED_EDGE ( 'NONE', *, *, #14271, .F. ) ;
#14318=FACE_OUTER_BOUND ( 'NONE', #35311, .T. ) ;
#14323=EDGE_CURVE ( 'NONE', #10821, #4637, #15941, .T. ) ;
#14367=EDGE_CURVE ( 'NONE', #30594, #5465, #1918, .T. ) ;
#14380=CARTESIAN_POINT ( 'NONE',  ( -44.00000000000000000, 0.000000000000000000, 0.000000000000000000 ) ) ;
#14395=EDGE_CURVE ( 'NONE', #16096, #12193, #5047, .T. ) ;
#14423=DIRECTION ( 'NONE',  ( -1.000000000000000000, -1.836970198721029934E-16, -0.000000000000000000 ) ) ;
#14426=ORIENTED_EDGE ( 'NONE', *, *, #25832, .F. ) ;
#14505=DIRECTION ( 'NONE',  ( -1.000000000000000000, -1.836970198721029934E-16, -0.000000000000000000 ) ) ;
#14525=EDGE_CURVE ( 'NONE', #4771, #4637, #6020, .T. ) ;
#14546=ADVANCED_FACE ( 'NONE', ( #3508 ), #5500, .F. ) ;
#14563=VERTEX_POINT ( 'NONE', #3154 ) ;
#14567=DIRECTION ( 'NONE',  ( 0.000000000000000000, -1.000000000000000000, 0.000000000000000000 ) ) ;
#14578=CARTESIAN_POINT ( 'NONE',  ( 23.00000000000000711, 4.000000000000005329, 4.898587196589404940E-16 ) ) ;
#14650=DIRECTION ( 'NONE',  ( 3.469446951953614682E-16, -1.000000000000000000, 0.000000000000000000 ) ) ;
#14670=DIRECTION ( 'NONE',  ( -1.000000000000000000, -1.836970198721029934E-16, -0.000000000000000000 ) ) ;
#14675=CARTESIAN_POINT ( 'NONE',  ( -29.99999999999999289, 2.571758278209443239E-15, 0.000000000000000000 ) ) ;
#14710=FACE_OUTER_BOUND ( 'NONE', #34640, .T. ) ;
#14736=ORIENTED_EDGE ( 'NONE', *, *, #8873, .T. ) ;
#14768=PLANE ( 'NONE',  #34694 ) ;
#14788=CIRCLE ( 'NONE', #33765, 11.00000000000000000 ) ;
#14874=CARTESIAN_POINT ( 'NONE',  ( 39.30000000000000426, 10.50000000000000355, 1.285879139104720436E-15 ) ) ;
#14897=ORIENTED_EDGE ( 'NONE', *, *, #19633, .T. ) ;
#14937=EDGE_LOOP ( 'NONE', ( #22987, #33870, #14297, #11383 ) ) ;
#15016=EDGE_CURVE ( 'NONE', #27829, #5432, #5979, .T. ) ;
#15052=DIRECTION ( 'NONE',  ( 0.000000000000000000, 0.000000000000000000, -1.000000000000000000 ) ) ;
#15056=FACE_OUTER_BOUND ( 'NONE', #165, .T. ) ;
#15065=AXIS2_PLACEMENT_3D ( 'NONE', #6357, #3675, #22914 ) ;
#15173=EDGE_CURVE ( 'NONE', #20385, #1882, #11563, .T. ) ;
#15190=( LENGTH_UNIT ( ) NAMED_UNIT ( * ) SI_UNIT ( .MILLI., .METRE. ) );
#15316=AXIS2_PLACEMENT_3D ( 'NONE', #2988, #8539, #11425 ) ;
#15469=EDGE_LOOP ( 'NONE', ( #33638, #9351 ) ) ;
#15476=ORIENTED_EDGE ( 'NONE', *, *, #11929, .T. ) ;
#15500=ORIENTED_EDGE ( 'NONE', *, *, #33042, .F. ) ;
#15515=CIRCLE ( 'NONE', #20108, 12.99999999999999467 ) ;
#15578=ORIENTED_EDGE ( 'NONE', *, *, #26164, .T. ) ;
#15592=CARTESIAN_POINT ( 'NONE',  ( -26.99999999999999289, 3.122849337825751800E-15, 0.000000000000000000 ) ) ;
#15608=VERTEX_POINT ( 'NONE', #6114 ) ;
#15704=DIRECTION ( 'NONE',  ( 0.000000000000000000, -1.000000000000000000, 0.000000000000000000 ) ) ;
#15727=DIRECTION ( 'NONE',  ( -1.000000000000000000, -1.836970198721029934E-16, -0.000000000000000000 ) ) ;
#15741=DIRECTION ( 'NONE',  ( -1.000000000000000000, -1.836970198721029934E-16, -0.000000000000000000 ) ) ;
#15749=ORIENTED_EDGE ( 'NONE', *, *, #14367, .T. ) ;
#15755=DIRECTION ( 'NONE',  ( 1.734723475976807834E-16, -1.000000000000000000, 0.000000000000000000 ) ) ;
#15868=DIRECTION ( 'NONE',  ( 0.000000000000000000, -1.000000000000000000, 0.000000000000000000 ) ) ;
#15941=CIRCLE ( 'NONE', #33704, 10.99999999999999822 ) ;
#15946=EDGE_LOOP ( 'NONE', ( #29203, #14426 ) ) ;
#15971=VERTEX_POINT ( 'NONE', #11473 ) ;
#16085=FACE_BOUND ( 'NONE', #6490, .T. ) ;
#16089=DIRECTION ( 'NONE',  ( -1.000000000000000000, -1.836970198721029934E-16, -0.000000000000000000 ) ) ;
#16096=VERTEX_POINT ( 'NONE', #14874 ) ;
#16109=ORIENTED_EDGE ( 'NONE', *, *, #34135, .F. ) ;
#16153=CARTESIAN_POINT ( 'NONE',  ( -43.99999999999999289, -45.00000000000000000, 0.000000000000000000 ) ) ;
#16186=AXIS2_PLACEMENT_3D ( 'NONE', #30093, #5085, #35330 ) ;
#16198=( GEOMETRIC_REPRESENTATION_CONTEXT ( 3 ) GLOBAL_UNCERTAINTY_ASSIGNED_CONTEXT ( ( #20769 ) ) GLOBAL_UNIT_ASSIGNED_CONTEXT ( ( #15190, #12702, #1358 ) ) REPRESENTATION_CONTEXT ( 'NONE', 'WORKASPACE' ) );
#16215=DIRECTION ( 'NONE',  ( -1.000000000000000000, -1.836970198721029934E-16, -0.000000000000000000 ) ) ;
#16236=CYLINDRICAL_SURFACE ( 'NONE', #30196, 3.999999999999998224 ) ;
#16254=PLANE ( 'NONE',  #4293 ) ;
#16262=FACE_BOUND ( 'NONE', #6165, .T. ) ;
#16270=DIRECTION ( 'NONE',  ( 1.000000000000000000, 1.836970198721029934E-16, 0.000000000000000000 ) ) ;
#16305=DIRECTION ( 'NONE',  ( -1.000000000000000000, -1.836970198721029934E-16, 0.000000000000000000 ) ) ;
#16349=SURFACE_SIDE_STYLE ('',( #30062 ) ) ;
#16356=EDGE_CURVE ( 'NONE', #12193, #16096, #17138, .T. ) ;
#16398=DIRECTION ( 'NONE',  ( -1.836970198721029934E-16, 1.000000000000000000, 0.000000000000000000 ) ) ;
#16450=CYLINDRICAL_SURFACE ( 'NONE', #17042, 3.999999999999993339 ) ;
#16472=EDGE_LOOP ( 'NONE', ( #16946, #8624, #16518, #5928, #4174 ) ) ;
#16476=DIRECTION ( 'NONE',  ( -1.000000000000000000, -1.836970198721029934E-16, -0.000000000000000000 ) ) ;
#16489=CIRCLE ( 'NONE', #8425, 19.99999999999999645 ) ;
#16518=ORIENTED_EDGE ( 'NONE', *, *, #6123, .T. ) ;
#16583=CARTESIAN_POINT ( 'NONE',  ( -26.99999999999999289, 3.122849337825751800E-15, 0.000000000000000000 ) ) ;
#16616=EDGE_CURVE ( 'NONE', #1882, #17302, #32140, .T. ) ;
#16695=ORIENTED_EDGE ( 'NONE', *, *, #33921, .T. ) ;
#16778=EDGE_LOOP ( 'NONE', ( #3291, #26670, #2246, #21114 ) ) ;
#16818=CIRCLE ( 'NONE', #3043, 44.99999999999999289 ) ;
#16834=EDGE_CURVE ( 'NONE', #1779, #41, #5654, .T. ) ;
#16897=CARTESIAN_POINT ( 'NONE',  ( 29.99999999999999645, 10.58300524425836819, 3.000000000000002665 ) ) ;
#16922=ORIENTED_EDGE ( 'NONE', *, *, #14395, .F. ) ;
#16944=DIRECTION ( 'NONE',  ( 0.000000000000000000, -1.000000000000000000, 0.000000000000000000 ) ) ;
#16946=ORIENTED_EDGE ( 'NONE', *, *, #16616, .T. ) ;
#16971=EDGE_CURVE ( 'NONE', #31067, #28461, #2279, .T. ) ;
#17013=DIRECTION ( 'NONE',  ( 1.541976423090495140E-16, -1.000000000000000000, 0.000000000000000000 ) ) ;
#17026=CARTESIAN_POINT ( 'NONE',  ( -44.00000000000000000, 1.349783804395672066E-31, 0.000000000000000000 ) ) ;
#17042=AXIS2_PLACEMENT_3D ( 'NONE', #21322, #18810, #21492 ) ;
#17068=CIRCLE ( 'NONE', #1652, 4.000000000000000000 ) ;
#17079=ORIENTED_EDGE ( 'NONE', *, *, #32873, .F. ) ;
#17132=DIRECTION ( 'NONE',  ( 0.000000000000000000, 0.000000000000000000, -1.000000000000000000 ) ) ;
#17138=CIRCLE ( 'NONE', #25808, 10.49999999999999645 ) ;
#17183=DIRECTION ( 'NONE',  ( -1.000000000000000000, -1.836970198721029934E-16, -0.000000000000000000 ) ) ;
#17207=EDGE_CURVE ( 'NONE', #24757, #10144, #4587, .T. ) ;
#17250=CARTESIAN_POINT ( 'NONE',  ( 27.00000000000000000, -19.99999999999997868, 0.000000000000000000 ) ) ;
#17279=CARTESIAN_POINT ( 'NONE',  ( -30.00000000000000355, 11.00000000000000000, 1.347111479062088405E-15 ) ) ;
#17302=VERTEX_POINT ( 'NONE', #34983 ) ;
#17400=CIRCLE ( 'NONE', #32384, 13.00000000000000000 ) ;
#17418=DIRECTION ( 'NONE',  ( 1.541976423090495140E-16, -1.000000000000000000, 0.000000000000000000 ) ) ;
#17433=EDGE_LOOP ( 'NONE', ( #18327, #8064, #1338, #22177 ) ) ;
#17439=ORIENTED_EDGE ( 'NONE', *, *, #25848, .T. ) ;
#17515=ORIENTED_EDGE ( 'NONE', *, *, #18033, .T. ) ;
#17536=LINE ( 'NONE', #284, #3045 ) ;
#17555=ORIENTED_EDGE ( 'NONE', *, *, #5363, .F. ) ;
#17575=CARTESIAN_POINT ( 'NONE',  ( -44.00199999999999534, -1.144142364505046046E-15, 3.000000000000002665 ) ) ;
#17588=DIRECTION ( 'NONE',  ( 1.000000000000000000, 1.836970198721029934E-16, 0.000000000000000000 ) ) ;
#17604=ORIENTED_EDGE ( 'NONE', *, *, #31775, .T. ) ;
#17750=( LENGTH_UNIT ( ) NAMED_UNIT ( * ) SI_UNIT ( .MILLI., .METRE. ) );
#17775=CARTESIAN_POINT ( 'NONE',  ( -29.99999999999999289, 2.571758278209443239E-15, 0.000000000000000000 ) ) ;
#17803=ADVANCED_FACE ( 'NONE', ( #15056, #1393 ), #12200, .F. ) ;
#17863=EDGE_CURVE ( 'NONE', #35305, #10821, #26967, .T. ) ;
#17876=ADVANCED_FACE ( 'NONE', ( #10215 ), #4471, .T. ) ;
#17893=CARTESIAN_POINT ( 'NONE',  ( -44.00000000000000000, 0.000000000000000000, 0.000000000000000000 ) ) ;
#17940=DIRECTION ( 'NONE',  ( -1.000000000000000000, -1.836970198721029934E-16, 0.000000000000000000 ) ) ;
#18020=VERTEX_POINT ( 'NONE', #7850 ) ;
#18033=EDGE_CURVE ( 'NONE', #6113, #35401, #35415, .T. ) ;
#18112=ORIENTED_EDGE ( 'NONE', *, *, #8873, .F. ) ;
#18181=DIRECTION ( 'NONE',  ( -1.000000000000000000, 0.000000000000000000, -0.000000000000000000 ) ) ;
#18268=LINE ( 'NONE', #12706, #2724 ) ;
#18290=AXIS2_PLACEMENT_3D ( 'NONE', #10421, #27161, #131 ) ;
#18292=DIRECTION ( 'NONE',  ( 1.000000000000000000, 0.000000000000000000, 0.000000000000000000 ) ) ;
#18327=ORIENTED_EDGE ( 'NONE', *, *, #8757, .F. ) ;
#18488=CIRCLE ( 'NONE', #30019, 3.999999999999994227 ) ;
#18533=ADVANCED_FACE ( 'NONE', ( #18575 ), #4911, .T. ) ;
#18569=DIRECTION ( 'NONE',  ( 0.000000000000000000, -1.000000000000000000, 0.000000000000000000 ) ) ;
#18575=FACE_OUTER_BOUND ( 'NONE', #27779, .T. ) ;
#18611=LINE ( 'NONE', #12689, #5896 ) ;
#18655=DIRECTION ( 'NONE',  ( -1.000000000000000000, -1.836970198721029934E-16, -0.000000000000000000 ) ) ;
#18659=DIRECTION ( 'NONE',  ( 1.000000000000000000, 1.836970198721029934E-16, 0.000000000000000000 ) ) ;
#18688=AXIS2_PLACEMENT_3D ( 'NONE', #24975, #11287, #30030 ) ;
#18706=DIRECTION ( 'NONE',  ( -1.000000000000000000, -1.836970198721029934E-16, -0.000000000000000000 ) ) ;
#18727=CARTESIAN_POINT ( 'NONE',  ( 44.00000000000000000, 11.00000000000001066, 1.347111479062088010E-15 ) ) ;
#18758=PLANE ( 'NONE',  #5905 ) ;
#18798=VECTOR ( 'NONE', #19290, 1000.000000000000000 ) ;
#18810=DIRECTION ( 'NONE',  ( -1.000000000000000000, -1.836970198721029934E-16, -0.000000000000000000 ) ) ;
#18873=ORIENTED_EDGE ( 'NONE', *, *, #28174, .F. ) ;
#18983=AXIS2_PLACEMENT_3D ( 'NONE', #5987, #28134, #16944 ) ;
#19050=CARTESIAN_POINT ( 'NONE',  ( -44.00000000000000000, -11.00000000000000000, 0.000000000000000000 ) ) ;
#19069=ORIENTED_EDGE ( 'NONE', *, *, #17863, .F. ) ;
#19100=VECTOR ( 'NONE', #22985, 1000.000000000000000 ) ;
#19138=AXIS2_PLACEMENT_3D ( 'NONE', #30888, #17183, #11445 ) ;
#19152=DIRECTION ( 'NONE',  ( -1.836970198721029934E-16, 1.000000000000000000, 0.000000000000000000 ) ) ;
#19290=DIRECTION ( 'NONE',  ( -1.000000000000000000, -1.836970198721029934E-16, -0.000000000000000000 ) ) ;
#19319=DIRECTION ( 'NONE',  ( 0.000000000000000000, -1.000000000000000000, 0.000000000000000000 ) ) ;
#19346=EDGE_LOOP ( 'NONE', ( #11566, #34409, #23129, #3627 ) ) ;
#19368=DIRECTION ( 'NONE',  ( -1.000000000000000000, -1.836970198721029934E-16, -0.000000000000000000 ) ) ;
#19404=AXIS2_PLACEMENT_3D ( 'NONE', #20143, #11180, #14567 ) ;
#19443=ORIENTED_EDGE ( 'NONE', *, *, #34135, .T. ) ;
#19502=FACE_OUTER_BOUND ( 'NONE', #13889, .T. ) ;
#19522=ADVANCED_FACE ( 'NONE', ( #26062 ), #1752, .F. ) ;
#19580=DIRECTION ( 'NONE',  ( -1.000000000000000000, -1.836970198721029934E-16, -0.000000000000000000 ) ) ;
#19633=EDGE_CURVE ( 'NONE', #24757, #12141, #7497, .T. ) ;
#19646=CYLINDRICAL_SURFACE ( 'NONE', #18983, 10.49999999999999645 ) ;
#19756=ORIENTED_EDGE ( 'NONE', *, *, #28725, .T. ) ;
#19760=EDGE_CURVE ( 'NONE', #12141, #4193, #28131, .T. ) ;
#19854=DIRECTION ( 'NONE',  ( 0.000000000000000000, -1.000000000000000000, 0.000000000000000000 ) ) ;
#19884=PLANE ( 'NONE',  #29629 ) ;
#19904=AXIS2_PLACEMENT_3D ( 'NONE', #25064, #14423, #14251 ) ;
#19922=FACE_BOUND ( 'NONE', #26951, .T. ) ;
#19967=DIRECTION ( 'NONE',  ( -1.000000000000000000, -1.836970198721029934E-16, -0.000000000000000000 ) ) ;
#19972=VECTOR ( 'NONE', #19967, 1000.000000000000000 ) ;
#20044=ORIENTED_EDGE ( 'NONE', *, *, #24243, .F. ) ;
#20052=AXIS2_PLACEMENT_3D ( 'NONE', #35072, #16476, #30181 ) ;
#20065=DIRECTION ( 'NONE',  ( -1.000000000000000000, -1.836970198721029934E-16, -0.000000000000000000 ) ) ;
#20090=VECTOR ( 'NONE', #24647, 1000.000000000000000 ) ;
#20106=LINE ( 'NONE', #28070, #1553 ) ;
#20108=AXIS2_PLACEMENT_3D ( 'NONE', #7722, #18706, #29706 ) ;
#20143=CARTESIAN_POINT ( 'NONE',  ( -44.00000000000000000, 0.000000000000000000, 0.000000000000000000 ) ) ;
#20196=MECHANICAL_DESIGN_GEOMETRIC_PRESENTATION_REPRESENTATION('',(#28866),#16198);
#20213=ORIENTED_EDGE ( 'NONE', *, *, #25848, .F. ) ;
#20242=DIRECTION ( 'NONE',  ( -1.000000000000000000, -1.836970198721029934E-16, -0.000000000000000000 ) ) ;
#20253=AXIS2_PLACEMENT_3D ( 'NONE', #14138, #808, #6223 ) ;
#20258=ORIENTED_EDGE ( 'NONE', *, *, #34308, .F. ) ;
#20271=DIRECTION ( 'NONE',  ( -0.000000000000000000, 0.000000000000000000, 1.000000000000000000 ) ) ;
#20331=ORIENTED_EDGE ( 'NONE', *, *, #31451, .T. ) ;
#20332=CARTESIAN_POINT ( 'NONE',  ( -44.00199999999999534, -1.144142364505046046E-15, -3.000000000000002665 ) ) ;
#20355=DIRECTION ( 'NONE',  ( -1.000000000000000000, -1.836970198721029934E-16, -0.000000000000000000 ) ) ;
#20385=VERTEX_POINT ( 'NONE', #22022 ) ;
#20417=CARTESIAN_POINT ( 'NONE',  ( -44.00000000000000000, 3.711905462088098291E-31, 0.000000000000000000 ) ) ;
#20436=SHAPE_DEFINITION_REPRESENTATION ( #1183, #27563 ) ;
#20466=DIRECTION ( 'NONE',  ( 1.541976423090495140E-16, -1.000000000000000000, 0.000000000000000000 ) ) ;
#20481=EDGE_LOOP ( 'NONE', ( #13431, #34591 ) ) ;
#20545=DIRECTION ( 'NONE',  ( -1.000000000000000000, -1.836970198721029934E-16, -0.000000000000000000 ) ) ;
#20625=ORIENTED_EDGE ( 'NONE', *, *, #14323, .F. ) ;
#20692=ORIENTED_EDGE ( 'NONE', *, *, #16834, .T. ) ;
#20720=DIRECTION ( 'NONE',  ( -1.000000000000000000, -1.836970198721029934E-16, -0.000000000000000000 ) ) ;
#20769=UNCERTAINTY_MEASURE_WITH_UNIT (LENGTH_MEASURE( 1.000000000000000082E-05 ), #15190, 'distance_accuracy_value', 'NONE');
#20843=VECTOR ( 'NONE', #9805, 1000.000000000000000 ) ;
#20844=AXIS2_PLACEMENT_3D ( 'NONE', #35135, #24319, #35309 ) ;
#20856=DIRECTION ( 'NONE',  ( 0.000000000000000000, 1.000000000000000000, 0.000000000000000000 ) ) ;
#20972=ORIENTED_EDGE ( 'NONE', *, *, #14271, .T. ) ;
#20984=AXIS2_PLACEMENT_3D ( 'NONE', #1012, #19580, #27717 ) ;
#21017=VERTEX_POINT ( 'NONE', #26971 ) ;
#21025=FACE_OUTER_BOUND ( 'NONE', #4634, .T. ) ;
#21071=CIRCLE ( 'NONE', #29736, 11.00000000000000000 ) ;
#21110=EDGE_CURVE ( 'NONE', #35305, #4771, #26044, .T. ) ;
#21113=ORIENTED_EDGE ( 'NONE', *, *, #16971, .F. ) ;
#21114=ORIENTED_EDGE ( 'NONE', *, *, #33323, .F. ) ;
#21126=EDGE_CURVE ( 'NONE', #28461, #31067, #150, .T. ) ;
#21174=EDGE_CURVE ( 'NONE', #1882, #15971, #17536, .T. ) ;
#21181=CARTESIAN_POINT ( 'NONE',  ( -44.00000000000000000, 0.000000000000000000, 0.000000000000000000 ) ) ;
#21285=EDGE_CURVE ( 'NONE', #33633, #31306, #1528, .T. ) ;
#21293=EDGE_LOOP ( 'NONE', ( #32427, #27895, #12255, #3351 ) ) ;
#21307=AXIS2_PLACEMENT_3D ( 'NONE', #26589, #12725, #18292 ) ;
#21322=CARTESIAN_POINT ( 'NONE',  ( -44.00000000000000000, 0.000000000000000000, 0.000000000000000000 ) ) ;
#21492=DIRECTION ( 'NONE',  ( 0.000000000000000000, -1.000000000000000000, 0.000000000000000000 ) ) ;
#21493=CARTESIAN_POINT ( 'NONE',  ( 29.99999999999999289, 1.244980450007031636E-14, 3.000000000000002665 ) ) ;
#21498=ORIENTED_EDGE ( 'NONE', *, *, #22194, .F. ) ;
#21657=CARTESIAN_POINT ( 'NONE',  ( -44.00000000000000000, 12.99999999999999822, 1.592040838891558898E-15 ) ) ;
#21658=LINE ( 'NONE', #31145, #31773 ) ;
#21671=CARTESIAN_POINT ( 'NONE',  ( 26.99999999999999289, 45.00000000000000711, 0.000000000000000000 ) ) ;
#21681=CARTESIAN_POINT ( 'NONE',  ( -30.00000000000000000, 2.571758278209441661E-15, 0.000000000000000000 ) ) ;
#21970=FACE_OUTER_BOUND ( 'NONE', #21293, .T. ) ;
#21988=FACE_OUTER_BOUND ( 'NONE', #29870, .T. ) ;
#22022=CARTESIAN_POINT ( 'NONE',  ( 37.99999999999999289, 10.58300524425836997, -3.000000000000002665 ) ) ;
#22043=FACE_OUTER_BOUND ( 'NONE', #14937, .T. ) ;
#22057=SHAPE_REPRESENTATION_RELATIONSHIP ( 'NONE' , 'NONE' ,  #27563, #9091 ) ;
#22177=ORIENTED_EDGE ( 'NONE', *, *, #13008, .F. ) ;
#22194=EDGE_CURVE ( 'NONE', #21017, #35346, #9572, .T. ) ;
#22196=UNCERTAINTY_MEASURE_WITH_UNIT (LENGTH_MEASURE( 1.000000000000000082E-05 ), #10200, 'distance_accuracy_value', 'NONE');
#22429=CARTESIAN_POINT ( 'NONE',  ( 30.00000000000000000, 1.359357947053562196E-14, 0.000000000000000000 ) ) ;
#22467=DIRECTION ( 'NONE',  ( 1.836970198721029934E-16, -1.000000000000000000, 0.000000000000000000 ) ) ;
#22487=EDGE_CURVE ( 'NONE', #21017, #32022, #25677, .T. ) ;
#22532=CARTESIAN_POINT ( 'NONE',  ( -44.00000000000000000, 10.58300524425835398, -3.000000000000002665 ) ) ;
#22543=MANIFOLD_SOLID_BREP ( 'Cut-Extrude-Thin1', #22711 ) ;
#22674=ADVANCED_FACE ( 'NONE', ( #16085, #32481 ), #5487, .F. ) ;
#22679=FACE_OUTER_BOUND ( 'NONE', #19346, .T. ) ;
#22711=CLOSED_SHELL ( 'NONE', ( #30595, #30415, #30643, #2540, #31364, #22891, #17876, #10784, #27234, #4650, #32619, #9222, #22674, #13333, #5768, #32217, #4814, #29554, #13018, #18533, #23200, #26191, #6437, #12111, #26205, #871, #34891, #17803, #19522, #14546, #1170, #8747, #4740 ) ) ;
#22714=ORIENTED_EDGE ( 'NONE', *, *, #35054, .F. ) ;
#22805=CARTESIAN_POINT ( 'NONE',  ( -44.00000000000000000, -4.000000000000000000, 0.000000000000000000 ) ) ;
#22852=DIRECTION ( 'NONE',  ( -1.000000000000000000, -1.836970198721029934E-16, -0.000000000000000000 ) ) ;
#22859=DIRECTION ( 'NONE',  ( 1.000000000000000000, 1.836970198721029934E-16, 0.000000000000000000 ) ) ;
#22891=ADVANCED_FACE ( 'NONE', ( #19502 ), #9062, .T. ) ;
#22894=ORIENTED_EDGE ( 'NONE', *, *, #3697, .T. ) ;
#22914=DIRECTION ( 'NONE',  ( 1.541976423090495387E-16, -1.000000000000000000, 0.000000000000000000 ) ) ;
#22985=DIRECTION ( 'NONE',  ( -1.000000000000000000, -1.836970198721029934E-16, -0.000000000000000000 ) ) ;
#22987=ORIENTED_EDGE ( 'NONE', *, *, #28230, .T. ) ;
#23052=ORIENTED_EDGE ( 'NONE', *, *, #15173, .F. ) ;
#23106=EDGE_CURVE ( 'NONE', #15608, #5432, #16818, .T. ) ;
#23129=ORIENTED_EDGE ( 'NONE', *, *, #32376, .T. ) ;
#23140=DIRECTION ( 'NONE',  ( 0.000000000000000000, -1.000000000000000000, 0.000000000000000000 ) ) ;
#23188=AXIS2_PLACEMENT_3D ( 'NONE', #24355, #16215, #2765 ) ;
#23200=ADVANCED_FACE ( 'NONE', ( #24531, #35520 ), #18758, .T. ) ;
#23211=VECTOR ( 'NONE', #13515, 1000.000000000000000 ) ;
#23418=DIRECTION ( 'NONE',  ( 0.000000000000000000, 0.000000000000000000, -1.000000000000000000 ) ) ;
#23434=ORIENTED_EDGE ( 'NONE', *, *, #14323, .T. ) ;
#23483=EDGE_CURVE ( 'NONE', #24879, #41, #17400, .T. ) ;
#23699=PRESENTATION_STYLE_ASSIGNMENT (( #12184 ) ) ;
#23800=ORIENTED_EDGE ( 'NONE', *, *, #1491, .T. ) ;
#23867=CIRCLE ( 'NONE', #20984, 13.00000000000000000 ) ;
#23871=ORIENTED_EDGE ( 'NONE', *, *, #26164, .F. ) ;
#23882=ORIENTED_EDGE ( 'NONE', *, *, #19760, .T. ) ;
#23933=CARTESIAN_POINT ( 'NONE',  ( -26.99999999999998934, -19.99999999999999289, 0.000000000000000000 ) ) ;
#24072=CYLINDRICAL_SURFACE ( 'NONE', #7612, 3.999999999999993339 ) ;
#24088=DIRECTION ( 'NONE',  ( 3.469446951953614682E-16, -1.000000000000000000, 0.000000000000000000 ) ) ;
#24160=CARTESIAN_POINT ( 'NONE',  ( 44.00000000000000000, 1.616533774874506480E-14, 0.000000000000000000 ) ) ;
#24186=AXIS2_PLACEMENT_3D ( 'NONE', #26326, #20545, #10102 ) ;
#24222=FACE_OUTER_BOUND ( 'NONE', #26907, .T. ) ;
#24243=EDGE_CURVE ( 'NONE', #34165, #20385, #7696, .T. ) ;
#24244=( NAMED_UNIT ( * ) PLANE_ANGLE_UNIT ( ) SI_UNIT ( $, .RADIAN. ) );
#24319=DIRECTION ( 'NONE',  ( -1.000000000000000000, -1.836970198721029934E-16, -0.000000000000000000 ) ) ;
#24336=ORIENTED_EDGE ( 'NONE', *, *, #25832, .T. ) ;
#24355=CARTESIAN_POINT ( 'NONE',  ( -44.00000000000000000, 0.000000000000000000, 0.000000000000000000 ) ) ;
#24365=PLANE ( 'NONE',  #25106 ) ;
#24389=DIRECTION ( 'NONE',  ( -1.000000000000000000, -1.836970198721030181E-16, 0.000000000000000000 ) ) ;
#24394=DIRECTION ( 'NONE',  ( 1.000000000000000000, 1.836970198721029934E-16, 0.000000000000000000 ) ) ;
#24402=CARTESIAN_POINT ( 'NONE',  ( 30.00000000000000000, 14.30000000000001315, 3.000000000000002665 ) ) ;
#24520=AXIS2_PLACEMENT_3D ( 'NONE', #22429, #3383, #11117 ) ;
#24531=FACE_BOUND ( 'NONE', #6282, .T. ) ;
#24554=CARTESIAN_POINT ( 'NONE',  ( -44.00000000000000000, 0.000000000000000000, 0.000000000000000000 ) ) ;
#24618=DIRECTION ( 'NONE',  ( -1.000000000000000000, -1.836970198721029934E-16, -0.000000000000000000 ) ) ;
#24623=VERTEX_POINT ( 'NONE', #24704 ) ;
#24644=ORIENTED_EDGE ( 'NONE', *, *, #9012, .T. ) ;
#24647=DIRECTION ( 'NONE',  ( -1.000000000000000000, -1.836970198721029934E-16, -0.000000000000000000 ) ) ;
#24693=AXIS2_PLACEMENT_3D ( 'NONE', #4203, #20355, #3841 ) ;
#24704=CARTESIAN_POINT ( 'NONE',  ( -29.99999999999999645, -10.99999999999999645, 0.000000000000000000 ) ) ;
#24757=VERTEX_POINT ( 'NONE', #6486 ) ;
#24779=STYLED_ITEM ( 'NONE', ( #23699 ), #9091 ) ;
#24782=ORIENTED_EDGE ( 'NONE', *, *, #28700, .T. ) ;
#24810=ORIENTED_EDGE ( 'NONE', *, *, #12636, .F. ) ;
#24853=VERTEX_POINT ( 'NONE', #17279 ) ;
#24876=DIRECTION ( 'NONE',  ( 1.541976423090495140E-16, -1.000000000000000000, 0.000000000000000000 ) ) ;
#24879=VERTEX_POINT ( 'NONE', #3991 ) ;
#24936=DIRECTION ( 'NONE',  ( -1.000000000000000000, -1.836970198721029934E-16, -0.000000000000000000 ) ) ;
#24941=DIRECTION ( 'NONE',  ( -1.000000000000000000, -1.836970198721029934E-16, -0.000000000000000000 ) ) ;
#24975=CARTESIAN_POINT ( 'NONE',  ( -44.00000000000000000, 0.000000000000000000, 0.000000000000000000 ) ) ;
#25064=CARTESIAN_POINT ( 'NONE',  ( 30.00000000000000000, 1.359357947053562196E-14, 0.000000000000000000 ) ) ;
#25106=AXIS2_PLACEMENT_3D ( 'NONE', #32645, #13555, #4588 ) ;
#25114=CARTESIAN_POINT ( 'NONE',  ( -44.00000000000000000, 0.000000000000000000, 0.000000000000000000 ) ) ;
#25123=VERTEX_POINT ( 'NONE', #32757 ) ;
#25165=AXIS2_PLACEMENT_3D ( 'NONE', #35050, #16270, #29456 ) ;
#25208=CARTESIAN_POINT ( 'NONE',  ( 22.99999999999998934, 13.00000000000000888, 1.592040838891559293E-15 ) ) ;
#25238=CARTESIAN_POINT ( 'NONE',  ( -23.00000000000000355, 4.000000000000000000, 4.898587196589411843E-16 ) ) ;
#25323=LINE ( 'NONE', #3188, #4994 ) ;
#25354=CARTESIAN_POINT ( 'NONE',  ( 38.00000000000000000, 1.391938065904714129E-14, -3.000000000000002665 ) ) ;
#25374=ORIENTED_EDGE ( 'NONE', *, *, #13008, .T. ) ;
#25386=DIRECTION ( 'NONE',  ( -1.000000000000000000, -1.836970198721029934E-16, -0.000000000000000000 ) ) ;
#25409=DIRECTION ( 'NONE',  ( 0.000000000000000000, -1.000000000000000000, 0.000000000000000000 ) ) ;
#25514=ORIENTED_EDGE ( 'NONE', *, *, #34, .T. ) ;
#25590=FACE_OUTER_BOUND ( 'NONE', #5685, .T. ) ;
#25619=CARTESIAN_POINT ( 'NONE',  ( 39.30000000000000426, 7.219292880973646134E-15, 0.000000000000000000 ) ) ;
#25677=LINE ( 'NONE', #9280, #31738 ) ;
#25693=DIRECTION ( 'NONE',  ( -1.000000000000000000, -1.836970198721029934E-16, -0.000000000000000000 ) ) ;
#25808=AXIS2_PLACEMENT_3D ( 'NONE', #25619, #14080, #17132 ) ;
#25825=PLANE ( 'NONE',  #30267 ) ;
#25832=EDGE_CURVE ( 'NONE', #5217, #27829, #7830, .T. ) ;
#25848=EDGE_CURVE ( 'NONE', #10144, #4193, #25323, .T. ) ;
#25931=( GEOMETRIC_REPRESENTATION_CONTEXT ( 3 ) GLOBAL_UNCERTAINTY_ASSIGNED_CONTEXT ( ( #22196 ) ) GLOBAL_UNIT_ASSIGNED_CONTEXT ( ( #10200, #24244, #10914 ) ) REPRESENTATION_CONTEXT ( 'NONE', 'WORKASPACE' ) );
#26016=DIRECTION ( 'NONE',  ( 3.154042683594196600E-16, -1.000000000000000000, 0.000000000000000000 ) ) ;
#26044=CIRCLE ( 'NONE', #19138, 10.99999999999999467 ) ;
#26061=CARTESIAN_POINT ( 'NONE',  ( 39.30000000000000426, -10.49999999999999112, 0.000000000000000000 ) ) ;
#26062=FACE_OUTER_BOUND ( 'NONE', #32067, .T. ) ;
#26075=CARTESIAN_POINT ( 'NONE',  ( 30.00000000000000000, 11.00000000000000711, 0.000000000000000000 ) ) ;
#26085=EDGE_CURVE ( 'NONE', #6113, #29440, #18268, .T. ) ;
#26164=EDGE_CURVE ( 'NONE', #24623, #24853, #9005, .T. ) ;
#26191=ADVANCED_FACE ( 'NONE', ( #24222 ), #16450, .F. ) ;
#26205=ADVANCED_FACE ( 'NONE', ( #16262, #32681 ), #8004, .T. ) ;
#26315=EDGE_LOOP ( 'NONE', ( #24644, #30254 ) ) ;
#26326=CARTESIAN_POINT ( 'NONE',  ( -44.00000000000000000, 0.000000000000000000, 0.000000000000000000 ) ) ;
#26376=EDGE_CURVE ( 'NONE', #5465, #4806, #28351, .T. ) ;
#26466=EDGE_CURVE ( 'NONE', #5432, #15608, #737, .T. ) ;
#26558=CARTESIAN_POINT ( 'NONE',  ( 30.00000000000000000, 1.359357947053562196E-14, 0.000000000000000000 ) ) ;
#26589=CARTESIAN_POINT ( 'NONE',  ( 0.000000000000000000, 0.000000000000000000, 0.000000000000000000 ) ) ;
#26590=AXIS2_PLACEMENT_3D ( 'NONE', #13412, #24394, #19152 ) ;
#26642=VERTEX_POINT ( 'NONE', #2723 ) ;
#26670=ORIENTED_EDGE ( 'NONE', *, *, #30199, .T. ) ;
#26710=CARTESIAN_POINT ( 'NONE',  ( 27.00000000000001066, 1.304248841091931379E-14, 0.000000000000000000 ) ) ;
#26733=DIRECTION ( 'NONE',  ( -1.000000000000000000, -1.836970198721029934E-16, -0.000000000000000000 ) ) ;
#26865=ORIENTED_EDGE ( 'NONE', *, *, #28230, .F. ) ;
#26907=EDGE_LOOP ( 'NONE', ( #2168, #29340, #15749, #13554 ) ) ;
#26929=CYLINDRICAL_SURFACE ( 'NONE', #28978, 10.99999999999999289 ) ;
#26951=EDGE_LOOP ( 'NONE', ( #5372, #34021 ) ) ;
#26967=LINE ( 'NONE', #13106, #31473 ) ;
#26971=CARTESIAN_POINT ( 'NONE',  ( -27.00000000000000000, 45.00000000000000000, 5.510910596163089556E-15 ) ) ;
#27127=AXIS2_PLACEMENT_3D ( 'NONE', #10598, #32030, #13139 ) ;
#27161=DIRECTION ( 'NONE',  ( -1.000000000000000000, -1.836970198721029934E-16, -0.000000000000000000 ) ) ;
#27172=DIRECTION ( 'NONE',  ( -1.000000000000000000, -1.836970198721029934E-16, -0.000000000000000000 ) ) ;
#27190=EDGE_CURVE ( 'NONE', #1275, #1779, #33070, .T. ) ;
#27234=ADVANCED_FACE ( 'NONE', ( #3023 ), #8574, .T. ) ;
#27250=FACE_BOUND ( 'NONE', #29561, .T. ) ;
#27276=CARTESIAN_POINT ( 'NONE',  ( -44.00000000000000000, -11.00000000000000000, 0.000000000000000000 ) ) ;
#27279=AXIS2_PLACEMENT_3D ( 'NONE', #7675, #18659, #4034 ) ;
#27284=CARTESIAN_POINT ( 'NONE',  ( 39.30000000000000426, 11.00000000000000533, 1.347111479062087419E-15 ) ) ;
#27436=CIRCLE ( 'NONE', #19904, 10.99999999999999289 ) ;
#27473=LINE ( 'NONE', #10904, #12402 ) ;
#27480=ORIENTED_EDGE ( 'NONE', *, *, #9791, .F. ) ;
#27563=SHAPE_REPRESENTATION ( 'winch drum', ( #21307 ), #35148 ) ;
#27593=DIRECTION ( 'NONE',  ( -1.000000000000000000, -1.836970198721029934E-16, -0.000000000000000000 ) ) ;
#27599=EDGE_CURVE ( 'NONE', #14563, #31368, #27473, .T. ) ;
#27717=DIRECTION ( 'NONE',  ( 2.668805347656626185E-16, -1.000000000000000000, 0.000000000000000000 ) ) ;
#27772=AXIS2_PLACEMENT_3D ( 'NONE', #30510, #8702, #429 ) ;
#27779=EDGE_LOOP ( 'NONE', ( #19069, #1513, #5924, #22894 ) ) ;
#27793=DIRECTION ( 'NONE',  ( 1.000000000000000000, 1.836970198721029934E-16, 0.000000000000000000 ) ) ;
#27829=VERTEX_POINT ( 'NONE', #31388 ) ;
#27840=DIRECTION ( 'NONE',  ( -1.836970198721029934E-16, 1.000000000000000000, 0.000000000000000000 ) ) ;
#27895=ORIENTED_EDGE ( 'NONE', *, *, #27190, .F. ) ;
#27929=ORIENTED_EDGE ( 'NONE', *, *, #26466, .F. ) ;
#27949=VECTOR ( 'NONE', #29047, 1000.000000000000000 ) ;
#27965=EDGE_CURVE ( 'NONE', #16096, #31067, #4584, .T. ) ;
#28070=CARTESIAN_POINT ( 'NONE',  ( 29.99999999999999289, 14.30000000000001315, 3.000000000000002665 ) ) ;
#28131=CIRCLE ( 'NONE', #20052, 4.000000000000000000 ) ;
#28134=DIRECTION ( 'NONE',  ( -1.000000000000000000, -1.836970198721030181E-16, 0.000000000000000000 ) ) ;
#28174=EDGE_CURVE ( 'NONE', #32022, #8923, #30248, .T. ) ;
#28187=AXIS2_PLACEMENT_3D ( 'NONE', #32684, #33036, #3152 ) ;
#28230=EDGE_CURVE ( 'NONE', #35346, #21017, #7843, .T. ) ;
#28240=VECTOR ( 'NONE', #27172, 1000.000000000000000 ) ;
#28285=CARTESIAN_POINT ( 'NONE',  ( 39.30000000000000426, 7.219292880973646134E-15, 0.000000000000000000 ) ) ;
#28300=ORIENTED_EDGE ( 'NONE', *, *, #27599, .T. ) ;
#28351=CIRCLE ( 'NONE', #27772, 3.999999999999993339 ) ;
#28461=VERTEX_POINT ( 'NONE', #13291 ) ;
#28507=CARTESIAN_POINT ( 'NONE',  ( 23.00000000000000000, 11.00000000000000533, 0.000000000000000000 ) ) ;
#28549=FILL_AREA_STYLE_COLOUR ( '', #12185 ) ;
#28563=CIRCLE ( 'NONE', #2141, 10.99999999999999822 ) ;
#28598=FACE_BOUND ( 'NONE', #16472, .T. ) ;
#28604=EDGE_LOOP ( 'NONE', ( #20044, #29733, #567, #23052 ) ) ;
#28655=ORIENTED_EDGE ( 'NONE', *, *, #34254, .T. ) ;
#28662=ORIENTED_EDGE ( 'NONE', *, *, #21174, .T. ) ;
#28700=EDGE_CURVE ( 'NONE', #18020, #30594, #9599, .T. ) ;
#28725=EDGE_CURVE ( 'NONE', #9377, #25123, #21071, .T. ) ;
#28771=PLANE ( 'NONE',  #29163 ) ;
#28775=CARTESIAN_POINT ( 'NONE',  ( 27.00000000000001776, -44.99999999999997868, 0.000000000000000000 ) ) ;
#28866=STYLED_ITEM ( 'NONE', ( #13678 ), #22543 ) ;
#28920=DIRECTION ( 'NONE',  ( 0.000000000000000000, -1.000000000000000000, 0.000000000000000000 ) ) ;
#28978=AXIS2_PLACEMENT_3D ( 'NONE', #34487, #15727, #2085 ) ;
#29047=DIRECTION ( 'NONE',  ( -1.000000000000000000, -1.836970198721030181E-16, 0.000000000000000000 ) ) ;
#29123=DIRECTION ( 'NONE',  ( -1.000000000000000000, -1.836970198721029934E-16, -0.000000000000000000 ) ) ;
#29158=AXIS2_PLACEMENT_3D ( 'NONE', #13773, #2981, #32485 ) ;
#29163=AXIS2_PLACEMENT_3D ( 'NONE', #9144, #680, #34002 ) ;
#29172=AXIS2_PLACEMENT_3D ( 'NONE', #7144, #17940, #20271 ) ;
#29203=ORIENTED_EDGE ( 'NONE', *, *, #14081, .F. ) ;
#29212=CYLINDRICAL_SURFACE ( 'NONE', #24186, 12.99999999999999822 ) ;
#29233=CIRCLE ( 'NONE', #18290, 10.99999999999999822 ) ;
#29264=CARTESIAN_POINT ( 'NONE',  ( 39.30000000000000426, -10.99999999999999112, 0.000000000000000000 ) ) ;
#29273=DIRECTION ( 'NONE',  ( -1.000000000000000000, -1.836970198721029934E-16, -0.000000000000000000 ) ) ;
#29340=ORIENTED_EDGE ( 'NONE', *, *, #11929, .F. ) ;
#29440=VERTEX_POINT ( 'NONE', #16897 ) ;
#29456=DIRECTION ( 'NONE',  ( 0.000000000000000000, 0.000000000000000000, -1.000000000000000000 ) ) ;
#29554=ADVANCED_FACE ( 'NONE', ( #3250 ), #534, .T. ) ;
#29561=EDGE_LOOP ( 'NONE', ( #6913, #16109 ) ) ;
#29585=DIRECTION ( 'NONE',  ( 1.541976423090495387E-16, -1.000000000000000000, 0.000000000000000000 ) ) ;
#29588=ORIENTED_EDGE ( 'NONE', *, *, #19633, .F. ) ;
#29629=AXIS2_PLACEMENT_3D ( 'NONE', #8569, #16305, #11455 ) ;
#29690=DIRECTION ( 'NONE',  ( -1.000000000000000000, -1.836970198721029934E-16, -0.000000000000000000 ) ) ;
#29706=DIRECTION ( 'NONE',  ( 2.668805347656627171E-16, -1.000000000000000000, 0.000000000000000000 ) ) ;
#29733=ORIENTED_EDGE ( 'NONE', *, *, #5363, .T. ) ;
#29736=AXIS2_PLACEMENT_3D ( 'NONE', #20417, #20242, #6760 ) ;
#29738=ORIENTED_EDGE ( 'NONE', *, *, #8229, .T. ) ;
#29743=CYLINDRICAL_SURFACE ( 'NONE', #16186, 12.99999999999999822 ) ;
#29870=EDGE_LOOP ( 'NONE', ( #20213, #14208, #14897, #23882 ) ) ;
#29874=CARTESIAN_POINT ( 'NONE',  ( -22.99999999999999645, 3.857637417314163478E-15, 0.000000000000000000 ) ) ;
#30000=EDGE_LOOP ( 'NONE', ( #15578, #23800, #6906, #17079 ) ) ;
#30019=AXIS2_PLACEMENT_3D ( 'NONE', #24160, #20720, #18569 ) ;
#30030=DIRECTION ( 'NONE',  ( 0.000000000000000000, -1.000000000000000000, 0.000000000000000000 ) ) ;
#30062=SURFACE_STYLE_FILL_AREA ( #3897 ) ;
#30092=CIRCLE ( 'NONE', #13406, 10.99999999999999822 ) ;
#30093=CARTESIAN_POINT ( 'NONE',  ( -44.00000000000000000, 0.000000000000000000, 0.000000000000000000 ) ) ;
#30143=UNCERTAINTY_MEASURE_WITH_UNIT (LENGTH_MEASURE( 1.000000000000000082E-05 ), #17750, 'distance_accuracy_value', 'NONE');
#30168=DIRECTION ( 'NONE',  ( -1.000000000000000000, -1.836970198721029934E-16, -0.000000000000000000 ) ) ;
#30181=DIRECTION ( 'NONE',  ( 0.000000000000000000, -1.000000000000000000, 0.000000000000000000 ) ) ;
#30196=AXIS2_PLACEMENT_3D ( 'NONE', #24554, #2786, #33004 ) ;
#30199=EDGE_CURVE ( 'NONE', #14563, #33633, #7206, .T. ) ;
#30237=CARTESIAN_POINT ( 'NONE',  ( -23.00000000000000000, 13.00000000000000533, 1.592040838891559293E-15 ) ) ;
#30248=CIRCLE ( 'NONE', #2092, 45.00000000000000000 ) ;
#30254=ORIENTED_EDGE ( 'NONE', *, *, #33323, .T. ) ;
#30267=AXIS2_PLACEMENT_3D ( 'NONE', #28507, #3861, #1149 ) ;
#30310=FACE_OUTER_BOUND ( 'NONE', #3108, .T. ) ;
#30316=DIRECTION ( 'NONE',  ( 1.000000000000000000, 1.836970198721029934E-16, 0.000000000000000000 ) ) ;
#30390=DIRECTION ( 'NONE',  ( 0.000000000000000000, -1.000000000000000000, 0.000000000000000000 ) ) ;
#30415=ADVANCED_FACE ( 'NONE', ( #30310 ), #16236, .F. ) ;
#30469=ORIENTED_EDGE ( 'NONE', *, *, #14367, .F. ) ;
#30476=CARTESIAN_POINT ( 'NONE',  ( -43.99999999999999289, -44.99999999999999289, 0.000000000000000000 ) ) ;
#30510=CARTESIAN_POINT ( 'NONE',  ( 23.00000000000000711, 1.230770033143090132E-14, 0.000000000000000000 ) ) ;
#30581=EDGE_CURVE ( 'NONE', #35401, #26642, #5647, .T. ) ;
#30594=VERTEX_POINT ( 'NONE', #8678 ) ;
#30595=ADVANCED_FACE ( 'NONE', ( #3654 ), #19646, .T. ) ;
#30615=ORIENTED_EDGE ( 'NONE', *, *, #21126, .F. ) ;
#30643=ADVANCED_FACE ( 'NONE', ( #4559 ), #29212, .F. ) ;
#30830=VECTOR ( 'NONE', #15741, 1000.000000000000000 ) ;
#30884=VECTOR ( 'NONE', #33971, 1000.000000000000000 ) ;
#30888=CARTESIAN_POINT ( 'NONE',  ( 44.00000000000000000, 1.616533774874506480E-14, 0.000000000000000000 ) ) ;
#30895=CARTESIAN_POINT ( 'NONE',  ( 30.00000000000000000, 1.359357947053562196E-14, 0.000000000000000000 ) ) ;
#30936=DIRECTION ( 'NONE',  ( 0.000000000000000000, 0.000000000000000000, -1.000000000000000000 ) ) ;
#30980=CARTESIAN_POINT ( 'NONE',  ( 44.00000000000000000, -10.99999999999997868, 0.000000000000000000 ) ) ;
#31012=ORIENTED_EDGE ( 'NONE', *, *, #30199, .F. ) ;
#31067=VERTEX_POINT ( 'NONE', #6294 ) ;
#31145=CARTESIAN_POINT ( 'NONE',  ( -44.00199999999999534, 14.29999999999999893, 3.000000000000002665 ) ) ;
#31306=VERTEX_POINT ( 'NONE', #23933 ) ;
#31361=ORIENTED_EDGE ( 'NONE', *, *, #8351, .F. ) ;
#31364=ADVANCED_FACE ( 'NONE', ( #21025 ), #8063, .T. ) ;
#31368=VERTEX_POINT ( 'NONE', #10429 ) ;
#31388=CARTESIAN_POINT ( 'NONE',  ( 30.00000000000000711, -44.99999999999997868, 0.000000000000000000 ) ) ;
#31451=EDGE_CURVE ( 'NONE', #35346, #8923, #7885, .T. ) ;
#31473=VECTOR ( 'NONE', #29123, 1000.000000000000000 ) ;
#31475=PLANE ( 'NONE',  #33369 ) ;
#31613=DIRECTION ( 'NONE',  ( -1.000000000000000000, -1.836970198721029934E-16, -0.000000000000000000 ) ) ;
#31641=DIRECTION ( 'NONE',  ( -1.000000000000000000, -1.836970198721029934E-16, -0.000000000000000000 ) ) ;
#31738=VECTOR ( 'NONE', #33581, 1000.000000000000000 ) ;
#31773=VECTOR ( 'NONE', #30316, 1000.000000000000000 ) ;
#31775=EDGE_CURVE ( 'NONE', #33633, #14563, #12171, .T. ) ;
#31971=CARTESIAN_POINT ( 'NONE',  ( -44.00000000000000000, 3.711905462088098291E-31, 0.000000000000000000 ) ) ;
#32022=VERTEX_POINT ( 'NONE', #32702 ) ;
#32030=DIRECTION ( 'NONE',  ( -1.000000000000000000, -1.836970198721029934E-16, -0.000000000000000000 ) ) ;
#32067=EDGE_LOOP ( 'NONE', ( #34104, #17515, #729, #34414 ) ) ;
#32140=CIRCLE ( 'NONE', #5699, 10.99999999999999289 ) ;
#32182=CARTESIAN_POINT ( 'NONE',  ( -29.99999999999998579, -45.00000000000000000, 0.000000000000000000 ) ) ;
#32202=PRODUCT_DEFINITION_FORMATION_WITH_SPECIFIED_SOURCE ( 'ANY', '', #1781, .NOT_KNOWN. ) ;
#32217=ADVANCED_FACE ( 'NONE', ( #12149 ), #11781, .T. ) ;
#32233=ORIENTED_EDGE ( 'NONE', *, *, #23106, .F. ) ;
#32253=COLOUR_RGB ( '', 0.66274510, 0.83137255, 0.94901961) ;
#32376=EDGE_CURVE ( 'NONE', #12193, #28461, #18611, .T. ) ;
#32384=AXIS2_PLACEMENT_3D ( 'NONE', #29874, #29690, #32922 ) ;
#32427=ORIENTED_EDGE ( 'NONE', *, *, #16834, .F. ) ;
#32481=FACE_OUTER_BOUND ( 'NONE', #7920, .T. ) ;
#32485=DIRECTION ( 'NONE',  ( -1.836970198721029934E-16, 1.000000000000000000, 0.000000000000000000 ) ) ;
#32579=ORIENTED_EDGE ( 'NONE', *, *, #26466, .T. ) ;
#32585=AXIS2_PLACEMENT_3D ( 'NONE', #21681, #16089, #2280 ) ;
#32592=EDGE_CURVE ( 'NONE', #10721, #35401, #21658, .T. ) ;
#32619=ADVANCED_FACE ( 'NONE', ( #894 ), #11874, .T. ) ;
#32645=CARTESIAN_POINT ( 'NONE',  ( -44.00000000000000000, 4.000000000000000000, 0.000000000000000000 ) ) ;
#32662=AXIS2_PLACEMENT_3D ( 'NONE', #14380, #25386, #700 ) ;
#32681=FACE_OUTER_BOUND ( 'NONE', #20481, .T. ) ;
#32684=CARTESIAN_POINT ( 'NONE',  ( -44.00000000000000000, 0.000000000000000000, 0.000000000000000000 ) ) ;
#32702=CARTESIAN_POINT ( 'NONE',  ( -30.00000000000000000, 45.00000000000000000, 5.510910596163089556E-15 ) ) ;
#32707=DIRECTION ( 'NONE',  ( -1.836970198721029934E-16, 1.000000000000000000, 0.000000000000000000 ) ) ;
#32735=AXIS2_PLACEMENT_3D ( 'NONE', #7986, #22852, #9174 ) ;
#32757=CARTESIAN_POINT ( 'NONE',  ( -44.00000000000000000, 11.00000000000000000, 1.347111479062088405E-15 ) ) ;
#32873=EDGE_CURVE ( 'NONE', #24623, #9377, #10259, .T. ) ;
#32922=DIRECTION ( 'NONE',  ( 2.668805347656626185E-16, -1.000000000000000000, 0.000000000000000000 ) ) ;
#33004=DIRECTION ( 'NONE',  ( 0.000000000000000000, -1.000000000000000000, 0.000000000000000000 ) ) ;
#33036=DIRECTION ( 'NONE',  ( -1.000000000000000000, -1.836970198721029934E-16, -0.000000000000000000 ) ) ;
#33040=ORIENTED_EDGE ( 'NONE', *, *, #21285, .F. ) ;
#33042=EDGE_CURVE ( 'NONE', #20385, #26642, #11648, .T. ) ;
#33068=FACE_OUTER_BOUND ( 'NONE', #12013, .T. ) ;
#33070=CIRCLE ( 'NONE', #2037, 12.99999999999999467 ) ;
#33229=ORIENTED_EDGE ( 'NONE', *, *, #14525, .F. ) ;
#33245=CYLINDRICAL_SURFACE ( 'NONE', #6734, 11.00000000000000000 ) ;
#33323=EDGE_CURVE ( 'NONE', #31368, #31306, #10234, .T. ) ;
#33369=AXIS2_PLACEMENT_3D ( 'NONE', #26075, #1406, #22467 ) ;
#33382=CARTESIAN_POINT ( 'NONE',  ( -44.00000000000000000, -10.99999999999999289, 0.000000000000000000 ) ) ;
#33413=FACE_BOUND ( 'NONE', #26315, .T. ) ;
#33523=DIRECTION ( 'NONE',  ( -1.000000000000000000, -1.836970198721029934E-16, -0.000000000000000000 ) ) ;
#33581=DIRECTION ( 'NONE',  ( -1.000000000000000000, -1.836970198721029934E-16, -0.000000000000000000 ) ) ;
#33597=ORIENTED_EDGE ( 'NONE', *, *, #3697, .F. ) ;
#33628=CARTESIAN_POINT ( 'NONE',  ( 29.99999999999999289, 45.00000000000000711, 5.510910596163087978E-15 ) ) ;
#33632=DIRECTION ( 'NONE',  ( -1.000000000000000000, -1.836970198721029934E-16, -0.000000000000000000 ) ) ;
#33633=VERTEX_POINT ( 'NONE', #17250 ) ;
#33638=ORIENTED_EDGE ( 'NONE', *, *, #8229, .F. ) ;
#33665=CARTESIAN_POINT ( 'NONE',  ( -44.00000000000000711, 44.99999999999999289, 5.510910596163087978E-15 ) ) ;
#33704=AXIS2_PLACEMENT_3D ( 'NONE', #12173, #34322, #1550 ) ;
#33730=VECTOR ( 'NONE', #24936, 1000.000000000000000 ) ;
#33759=DIRECTION ( 'NONE',  ( -1.000000000000000000, -1.836970198721029934E-16, -0.000000000000000000 ) ) ;
#33765=AXIS2_PLACEMENT_3D ( 'NONE', #31971, #31613, #28920 ) ;
#33779=DIRECTION ( 'NONE',  ( -1.000000000000000000, -1.836970198721029934E-16, -0.000000000000000000 ) ) ;
#33870=ORIENTED_EDGE ( 'NONE', *, *, #22487, .T. ) ;
#33921=EDGE_CURVE ( 'NONE', #24853, #24623, #29233, .T. ) ;
#33971=DIRECTION ( 'NONE',  ( -1.000000000000000000, -1.836970198721029934E-16, -0.000000000000000000 ) ) ;
#34002=DIRECTION ( 'NONE',  ( -1.836970198721029934E-16, 1.000000000000000000, 0.000000000000000000 ) ) ;
#34003=CARTESIAN_POINT ( 'NONE',  ( -44.00199999999999534, 14.29999999999999893, -3.000000000000002665 ) ) ;
#34019=ORIENTED_EDGE ( 'NONE', *, *, #18033, .F. ) ;
#34021=ORIENTED_EDGE ( 'NONE', *, *, #14395, .T. ) ;
#34104=ORIENTED_EDGE ( 'NONE', *, *, #26085, .F. ) ;
#34135=EDGE_CURVE ( 'NONE', #4193, #12141, #17068, .T. ) ;
#34147=CARTESIAN_POINT ( 'NONE',  ( -44.00000000000000000, 3.999999999999993339, 4.898587196589404940E-16 ) ) ;
#34165=VERTEX_POINT ( 'NONE', #653 ) ;
#34181=CARTESIAN_POINT ( 'NONE',  ( -44.00000000000000000, -10.99999999999999289, 0.000000000000000000 ) ) ;
#34254=EDGE_CURVE ( 'NONE', #18020, #4806, #9470, .T. ) ;
#34268=FACE_BOUND ( 'NONE', #9878, .T. ) ;
#34308=EDGE_CURVE ( 'NONE', #25123, #9377, #14788, .T. ) ;
#34322=DIRECTION ( 'NONE',  ( 1.000000000000000000, 1.836970198721029934E-16, 0.000000000000000000 ) ) ;
#34358=AXIS2_PLACEMENT_3D ( 'NONE', #21181, #18655, #24088 ) ;
#34365=AXIS2_PLACEMENT_3D ( 'NONE', #14675, #9653, #9295 ) ;
#34372=ORIENTED_EDGE ( 'NONE', *, *, #30581, .F. ) ;
#34409=ORIENTED_EDGE ( 'NONE', *, *, #16356, .F. ) ;
#34414=ORIENTED_EDGE ( 'NONE', *, *, #6123, .F. ) ;
#34487=CARTESIAN_POINT ( 'NONE',  ( -44.00000000000000000, 0.000000000000000000, 0.000000000000000000 ) ) ;
#34511=FILL_AREA_STYLE ('',( #10013 ) ) ;
#34591=ORIENTED_EDGE ( 'NONE', *, *, #34, .F. ) ;
#34640=EDGE_LOOP ( 'NONE', ( #33597, #20625 ) ) ;
#34694=AXIS2_PLACEMENT_3D ( 'NONE', #20332, #23418, #18181 ) ;
#34697=CARTESIAN_POINT ( 'NONE',  ( 26.99999999999999645, 1.304248841091931221E-14, 0.000000000000000000 ) ) ;
#34818=DIRECTION ( 'NONE',  ( -1.000000000000000000, -1.836970198721029934E-16, -0.000000000000000000 ) ) ;
#34832=EDGE_CURVE ( 'NONE', #10144, #24757, #9003, .T. ) ;
#34891=ADVANCED_FACE ( 'NONE', ( #35007, #27250 ), #24365, .T. ) ;
#34964=EDGE_LOOP ( 'NONE', ( #13093, #31012 ) ) ;
#34983=CARTESIAN_POINT ( 'NONE',  ( 30.00000000000000355, -10.99999999999997868, 0.000000000000000000 ) ) ;
#35007=FACE_OUTER_BOUND ( 'NONE', #4344, .T. ) ;
#35020=ORIENTED_EDGE ( 'NONE', *, *, #26376, .F. ) ;
#35050=CARTESIAN_POINT ( 'NONE',  ( 39.30000000000000426, 7.219292880973646134E-15, 0.000000000000000000 ) ) ;
#35054=EDGE_CURVE ( 'NONE', #17302, #29440, #27436, .T. ) ;
#35072=CARTESIAN_POINT ( 'NONE',  ( -44.00000000000000000, 1.349783804395672066E-31, 0.000000000000000000 ) ) ;
#35135=CARTESIAN_POINT ( 'NONE',  ( 27.00000000000001066, 1.304248841091931379E-14, 0.000000000000000000 ) ) ;
#35148=( GEOMETRIC_REPRESENTATION_CONTEXT ( 3 ) GLOBAL_UNCERTAINTY_ASSIGNED_CONTEXT ( ( #30143 ) ) GLOBAL_UNIT_ASSIGNED_CONTEXT ( ( #17750, #1739, #6955 ) ) REPRESENTATION_CONTEXT ( 'NONE', 'WORKASPACE' ) );
#35173=CYLINDRICAL_SURFACE ( 'NONE', #23188, 3.999999999999998224 ) ;
#35272=ORIENTED_EDGE ( 'NONE', *, *, #14081, .T. ) ;
#35305=VERTEX_POINT ( 'NONE', #18727 ) ;
#35309=DIRECTION ( 'NONE',  ( 1.541976423090495387E-16, -1.000000000000000000, 0.000000000000000000 ) ) ;
#35311=EDGE_LOOP ( 'NONE', ( #26865, #21498 ) ) ;
#35330=DIRECTION ( 'NONE',  ( 0.000000000000000000, -1.000000000000000000, 0.000000000000000000 ) ) ;
#35346=VERTEX_POINT ( 'NONE', #13347 ) ;
#35389=CYLINDRICAL_SURFACE ( 'NONE', #28187, 45.00000000000000000 ) ;
#35401=VERTEX_POINT ( 'NONE', #9920 ) ;
#35415=LINE ( 'NONE', #10744, #35522 ) ;
#35520=FACE_OUTER_BOUND ( 'NONE', #15469, .T. ) ;
#35522=VECTOR ( 'NONE', #32707, 1000.000000000000000 ) ;
ENDSEC;
END-ISO-10303-21;
